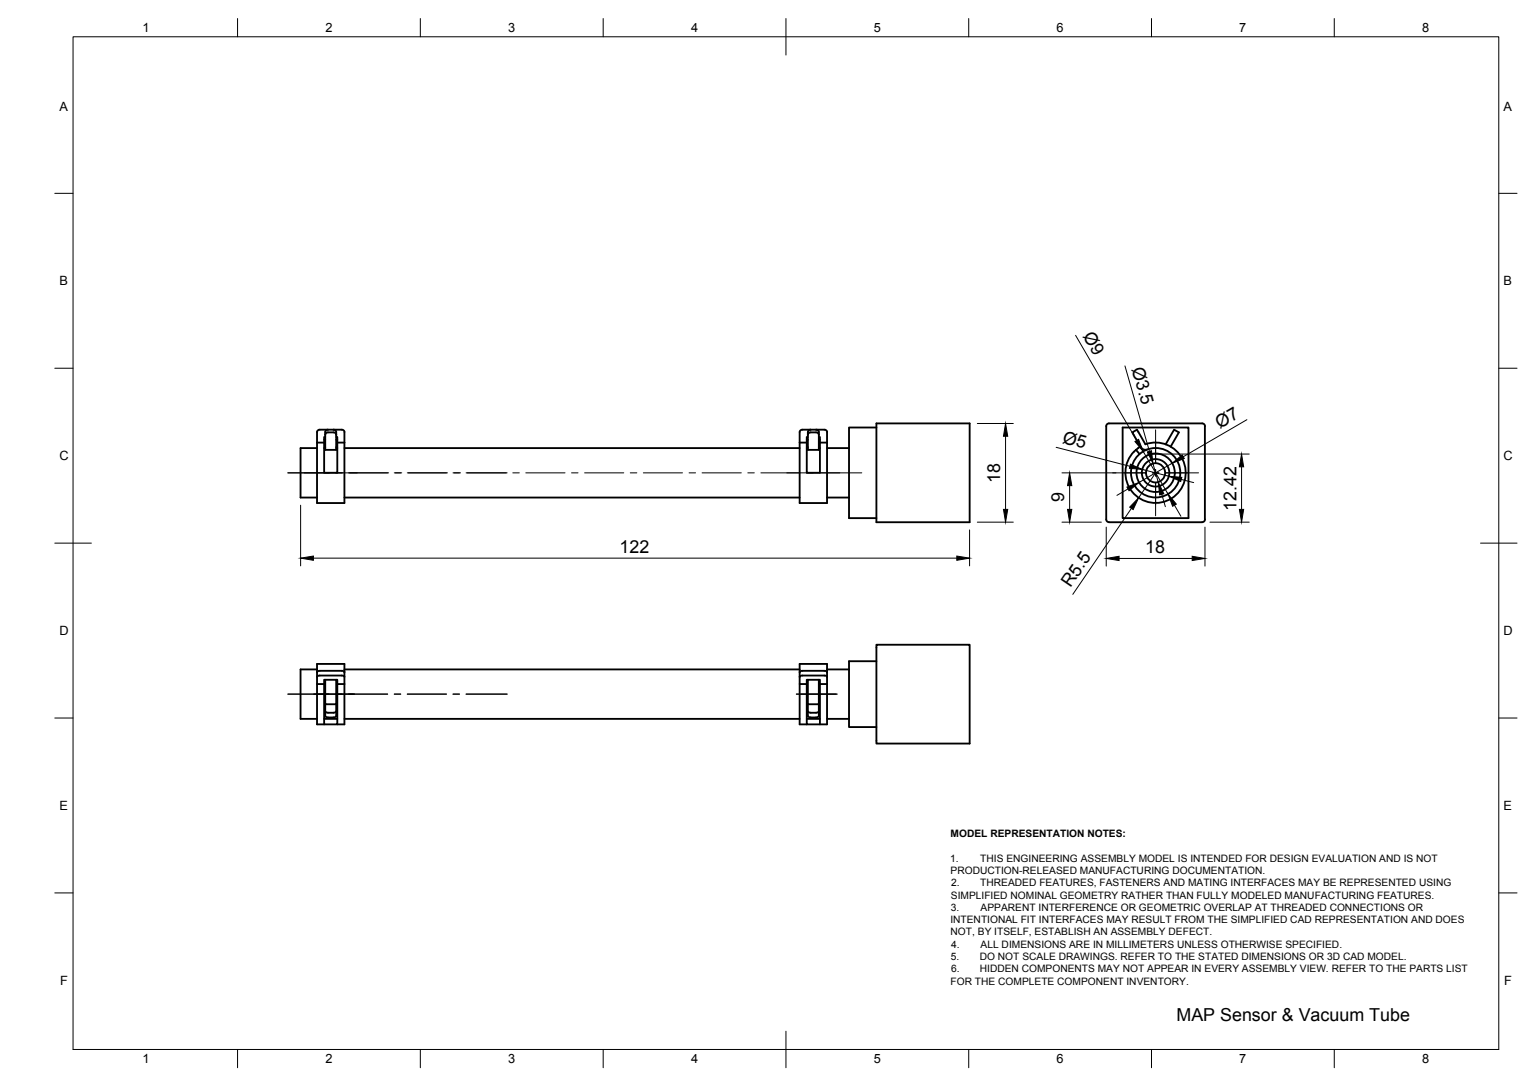
ISO-10303-21;
HEADER;
/* Generated by software containing ST-Developer
 * from STEP Tools, Inc. (www.steptools.com) 
 */

FILE_DESCRIPTION(
/* description */ ('STEP AP214'),
/* implementation_level */ '2;1');

FILE_NAME(
/* name */ 'MAP Sensor & Vacuum Tube.step',
/* time_stamp */ '2026-10-07T12:18:07-07:00',
/* author */ (''),
/* organization */ (''),
/* preprocessor_version */ 'ST-DEVELOPER v20.2',
/* originating_system */ 'Autodesk Translation Framework v15.15.0.0',
/* authorisation */ '');

FILE_SCHEMA (('AUTOMOTIVE_DESIGN { 1 0 10303 214 3 1 1 }'));
ENDSEC;

DATA;
#10=MECHANICAL_DESIGN_GEOMETRIC_PRESENTATION_REPRESENTATION('',(#128),#62974);
#104=SHAPE_REPRESENTATION_RELATIONSHIP('SRR','None',#63027,#116);
#116=ADVANCED_BREP_SHAPE_REPRESENTATION('',(#140),#62968);
#128=STYLED_ITEM('',(#63090),#140);
#140=MANIFOLD_SOLID_BREP('Body1',#15198);
#234=FACE_BOUND('',#5113,.T.);
#235=FACE_BOUND('',#5164,.T.);
#236=FACE_BOUND('',#5166,.T.);
#237=FACE_BOUND('',#5176,.T.);
#238=FACE_BOUND('',#5179,.T.);
#239=FACE_BOUND('',#5183,.T.);
#589=PLANE('',#16296);
#590=PLANE('',#16297);
#591=PLANE('',#16298);
#592=PLANE('',#16302);
#593=PLANE('',#16303);
#594=PLANE('',#16306);
#595=PLANE('',#16311);
#596=PLANE('',#16312);
#597=PLANE('',#16313);
#598=PLANE('',#16315);
#599=PLANE('',#16316);
#600=PLANE('',#16320);
#601=PLANE('',#16321);
#602=PLANE('',#16323);
#603=PLANE('',#16324);
#604=PLANE('',#16325);
#605=PLANE('',#16327);
#606=PLANE('',#16329);
#607=PLANE('',#16333);
#608=PLANE('',#16334);
#609=PLANE('',#16336);
#610=PLANE('',#16337);
#611=PLANE('',#16338);
#612=PLANE('',#16340);
#613=PLANE('',#16341);
#614=PLANE('',#16342);
#615=PLANE('',#16344);
#616=PLANE('',#16345);
#617=PLANE('',#16349);
#618=PLANE('',#16350);
#619=PLANE('',#16357);
#620=PLANE('',#16358);
#621=PLANE('',#16360);
#622=PLANE('',#16361);
#623=PLANE('',#16362);
#624=PLANE('',#16363);
#625=PLANE('',#16364);
#626=PLANE('',#16365);
#627=PLANE('',#16366);
#628=PLANE('',#16367);
#629=PLANE('',#16371);
#630=PLANE('',#16375);
#631=PLANE('',#16376);
#632=PLANE('',#16381);
#633=PLANE('',#16383);
#634=PLANE('',#16384);
#635=PLANE('',#16385);
#636=PLANE('',#16386);
#896=B_SPLINE_CURVE_WITH_KNOTS('',3,(#44539,#44540,#44541,#44542,#44543,
#44544,#44545,#44546,#44547,#44548),.UNSPECIFIED.,.F.,.F.,(4,2,2,2,4),(0.22713486148052,
0.24601821426655,0.264901567052579,0.283737456690072,0.302573346327564),
 .UNSPECIFIED.);
#897=B_SPLINE_CURVE_WITH_KNOTS('',3,(#44552,#44553,#44554,#44555,#44556,
#44557,#44558,#44559,#44560,#44561),.UNSPECIFIED.,.F.,.F.,(4,2,2,2,4),(-0.151286623693373,
-0.132450734062243,-0.113614844431112,-0.0947314916401544,-0.0758481388491969),
 .UNSPECIFIED.);
#898=B_SPLINE_CURVE_WITH_KNOTS('',3,(#44593,#44594,#44595,#44596,#44597,
#44598,#44599,#44600,#44601,#44602),.UNSPECIFIED.,.F.,.F.,(4,2,2,2,4),(0.227134861433275,
0.246018214232104,0.264901567030932,0.283737456679245,0.302573346327559),
 .UNSPECIFIED.);
#899=B_SPLINE_CURVE_WITH_KNOTS('',3,(#44606,#44607,#44608,#44609,#44610,
#44611,#44612,#44613,#44614,#44615),.UNSPECIFIED.,.F.,.F.,(4,2,2,2,4),(-0.151286623693374,
-0.132450734061232,-0.113614844429089,-0.0947314916371198,-0.0758481388451503),
 .UNSPECIFIED.);
#900=B_SPLINE_CURVE_WITH_KNOTS('',3,(#44623,#44624,#44625,#44626,#44627,
#44628,#44629,#44630,#44631,#44632),.UNSPECIFIED.,.F.,.F.,(4,2,2,2,4),(-0.075438484844178,
-0.0565551320532202,-0.0376717792622623,-0.0188358896311301,2.13717932240343E-15),
 .UNSPECIFIED.);
#901=B_SPLINE_CURVE_WITH_KNOTS('',3,(#44636,#44637,#44638,#44639,#44640,
#44641,#44642,#44643,#44644,#44645),.UNSPECIFIED.,.F.,.F.,(4,2,2,2,4),(1.23169706186427E-15,
0.0188358896365198,0.0376717792730385,0.056555132060041,0.0754384848470435),
 .UNSPECIFIED.);
#902=B_SPLINE_CURVE_WITH_KNOTS('',3,(#44665,#44666,#44667,#44668,#44669,
#44670,#44671,#44672,#44673,#44674),.UNSPECIFIED.,.F.,.F.,(4,2,2,2,4),(-0.075438484902782,
-0.0565551320981278,-0.0376717792934735,-0.0188358896467368,0.),
 .UNSPECIFIED.);
#903=B_SPLINE_CURVE_WITH_KNOTS('',3,(#44678,#44679,#44680,#44681,#44682,
#44683,#44684,#44685,#44686,#44687),.UNSPECIFIED.,.F.,.F.,(4,2,2,2,4),(-2.21579007906029E-15,
0.01883588963867,0.0376717792773423,0.0565551320645541,0.0754384848517659),
 .UNSPECIFIED.);
#904=B_SPLINE_CURVE_WITH_KNOTS('',3,(#44704,#44705,#44706,#44707,#44708,
#44709,#44710,#44711,#44712,#44713),.UNSPECIFIED.,.F.,.F.,(4,2,2,2,4),(0.226757476774398,
0.245624555668826,0.264491634563253,0.283327009974748,0.302162385386242),
 .UNSPECIFIED.);
#905=B_SPLINE_CURVE_WITH_KNOTS('',3,(#44717,#44718,#44719,#44720,#44721,
#44722,#44723,#44724,#44725,#44726),.UNSPECIFIED.,.F.,.F.,(4,2,2,2,4),(-0.15108117139346,
-0.132245795981966,-0.113410420570472,-0.0945433416760444,-0.0756762627816166),
 .UNSPECIFIED.);
#906=B_SPLINE_CURVE_WITH_KNOTS('',3,(#44734,#44735,#44736,#44737,#44738,
#44739,#44740,#44741,#44742,#44743),.UNSPECIFIED.,.F.,.F.,(4,2,2,2,4),(-0.226486122604629,
-0.207619043710201,-0.188751964815772,-0.169916589404278,-0.151081213992783),
 .UNSPECIFIED.);
#907=B_SPLINE_CURVE_WITH_KNOTS('',3,(#44747,#44748,#44749,#44750,#44751,
#44752,#44753,#44754,#44755,#44756),.UNSPECIFIED.,.F.,.F.,(4,2,2,2,4),(0.151081213992781,
0.169916589404275,0.18875196481577,0.207619043710198,0.226486122604627),
 .UNSPECIFIED.);
#908=B_SPLINE_CURVE_WITH_KNOTS('',3,(#44765,#44766,#44767,#44768,#44769,
#44770,#44771,#44772,#44773,#44774),.UNSPECIFIED.,.F.,.F.,(4,2,2,2,4),(0.226757476774397,
0.245624555668825,0.264491634563252,0.283327009974748,0.302162385386243),
 .UNSPECIFIED.);
#909=B_SPLINE_CURVE_WITH_KNOTS('',3,(#44778,#44779,#44780,#44781,#44782,
#44783,#44784,#44785,#44786,#44787),.UNSPECIFIED.,.F.,.F.,(4,2,2,2,4),(-0.151081213992782,
-0.132245838581287,-0.113410463169793,-0.0945433842753652,-0.0756763053809372),
 .UNSPECIFIED.);
#910=B_SPLINE_CURVE_WITH_KNOTS('',3,(#44795,#44796,#44797,#44798,#44799,
#44800,#44801,#44802,#44803,#44804),.UNSPECIFIED.,.F.,.F.,(4,2,2,2,4),(-0.226486080005305,
-0.207619001110877,-0.188751922216448,-0.169916546804955,-0.151081171393461),
 .UNSPECIFIED.);
#911=B_SPLINE_CURVE_WITH_KNOTS('',3,(#44808,#44809,#44810,#44811,#44812,
#44813,#44814,#44815,#44816,#44817),.UNSPECIFIED.,.F.,.F.,(4,2,2,2,4),(0.151081171393462,
0.169916546804955,0.188751922216448,0.207619001110876,0.226486080005304),
 .UNSPECIFIED.);
#1803=LINE('',#44535,#2996);
#1804=LINE('',#44550,#2997);
#1805=LINE('',#44565,#2998);
#1806=LINE('',#44570,#2999);
#1807=LINE('',#44575,#3000);
#1808=LINE('',#44579,#3001);
#1809=LINE('',#44584,#3002);
#1810=LINE('',#44589,#3003);
#1811=LINE('',#44604,#3004);
#1812=LINE('',#44619,#3005);
#1813=LINE('',#44634,#3006);
#1814=LINE('',#44650,#3007);
#1815=LINE('',#44655,#3008);
#1816=LINE('',#44661,#3009);
#1817=LINE('',#44676,#3010);
#1818=LINE('',#44691,#3011);
#1819=LINE('',#44695,#3012);
#1820=LINE('',#44700,#3013);
#1821=LINE('',#44715,#3014);
#1822=LINE('',#44730,#3015);
#1823=LINE('',#44745,#3016);
#1824=LINE('',#44761,#3017);
#1825=LINE('',#44776,#3018);
#1826=LINE('',#44791,#3019);
#1827=LINE('',#44806,#3020);
#1828=LINE('',#44823,#3021);
#1829=LINE('',#44829,#3022);
#1830=LINE('',#44835,#3023);
#1831=LINE('',#44842,#3024);
#1832=LINE('',#44845,#3025);
#1833=LINE('',#44850,#3026);
#1834=LINE('',#44856,#3027);
#1835=LINE('',#44862,#3028);
#1836=LINE('',#44866,#3029);
#1837=LINE('',#44870,#3030);
#1838=LINE('',#44876,#3031);
#1839=LINE('',#44882,#3032);
#1840=LINE('',#44888,#3033);
#1841=LINE('',#44892,#3034);
#1842=LINE('',#44896,#3035);
#1843=LINE('',#44903,#3036);
#1844=LINE('',#44908,#3037);
#1845=LINE('',#44916,#3038);
#1846=LINE('',#44920,#3039);
#1847=LINE('',#44921,#3040);
#1848=LINE('',#44923,#3041);
#1849=LINE('',#44924,#3042);
#1850=LINE('',#44930,#3043);
#1851=LINE('',#44933,#3044);
#1852=LINE('',#44935,#3045);
#1853=LINE('',#44936,#3046);
#1854=LINE('',#44937,#3047);
#1855=LINE('',#44940,#3048);
#1856=LINE('',#44943,#3049);
#1857=LINE('',#44946,#3050);
#1858=LINE('',#44948,#3051);
#1859=LINE('',#44950,#3052);
#1860=LINE('',#44951,#3053);
#1861=LINE('',#44954,#3054);
#1862=LINE('',#44957,#3055);
#1863=LINE('',#44959,#3056);
#1864=LINE('',#44961,#3057);
#1865=LINE('',#44964,#3058);
#1866=LINE('',#44966,#3059);
#1867=LINE('',#44967,#3060);
#1868=LINE('',#44969,#3061);
#1869=LINE('',#44970,#3062);
#1870=LINE('',#44975,#3063);
#1871=LINE('',#44976,#3064);
#1872=LINE('',#44981,#3065);
#1873=LINE('',#44985,#3066);
#1874=LINE('',#44987,#3067);
#1875=LINE('',#44988,#3068);
#1876=LINE('',#44992,#3069);
#1877=LINE('',#44994,#3070);
#1878=LINE('',#44995,#3071);
#1879=LINE('',#44998,#3072);
#1880=LINE('',#45000,#3073);
#1881=LINE('',#45001,#3074);
#1882=LINE('',#45003,#3075);
#1883=LINE('',#45006,#3076);
#1884=LINE('',#45010,#3077);
#1885=LINE('',#45011,#3078);
#1886=LINE('',#45017,#3079);
#1887=LINE('',#45020,#3080);
#1888=LINE('',#45023,#3081);
#1889=LINE('',#45025,#3082);
#1890=LINE('',#45026,#3083);
#1891=LINE('',#45030,#3084);
#1892=LINE('',#45032,#3085);
#1893=LINE('',#45034,#3086);
#1894=LINE('',#45035,#3087);
#1895=LINE('',#45036,#3088);
#1896=LINE('',#45039,#3089);
#1897=LINE('',#45041,#3090);
#1898=LINE('',#45042,#3091);
#1899=LINE('',#45044,#3092);
#1900=LINE('',#45047,#3093);
#1901=LINE('',#45049,#3094);
#1902=LINE('',#45050,#3095);
#1903=LINE('',#45052,#3096);
#1904=LINE('',#45053,#3097);
#1905=LINE('',#45055,#3098);
#1906=LINE('',#45059,#3099);
#1907=LINE('',#45060,#3100);
#1908=LINE('',#45062,#3101);
#1909=LINE('',#45063,#3102);
#1910=LINE('',#45069,#3103);
#1911=LINE('',#45072,#3104);
#1912=LINE('',#45074,#3105);
#1913=LINE('',#45075,#3106);
#1914=LINE('',#45076,#3107);
#1915=LINE('',#45079,#3108);
#1916=LINE('',#45082,#3109);
#1917=LINE('',#45086,#3110);
#1918=LINE('',#45089,#3111);
#1919=LINE('',#45091,#3112);
#1920=LINE('',#45094,#3113);
#1921=LINE('',#45095,#3114);
#1922=LINE('',#45106,#3115);
#1923=LINE('',#45108,#3116);
#1924=LINE('',#45110,#3117);
#1925=LINE('',#45111,#3118);
#1926=LINE('',#45114,#3119);
#1927=LINE('',#45116,#3120);
#1928=LINE('',#45117,#3121);
#1929=LINE('',#45121,#3122);
#1930=LINE('',#45123,#3123);
#1931=LINE('',#45125,#3124);
#1932=LINE('',#45126,#3125);
#1933=LINE('',#45131,#3126);
#1934=LINE('',#45135,#3127);
#1935=LINE('',#45137,#3128);
#1936=LINE('',#45138,#3129);
#1937=LINE('',#45143,#3130);
#1938=LINE('',#45147,#3131);
#1939=LINE('',#45149,#3132);
#1940=LINE('',#45150,#3133);
#1941=LINE('',#45155,#3134);
#1942=LINE('',#45159,#3135);
#1943=LINE('',#45163,#3136);
#1944=LINE('',#45166,#3137);
#1945=LINE('',#45167,#3138);
#1946=LINE('',#45169,#3139);
#1947=LINE('',#45172,#3140);
#1948=LINE('',#45173,#3141);
#1949=LINE('',#45175,#3142);
#2996=VECTOR('',#19460,4.5);
#2997=VECTOR('',#19463,1000.);
#2998=VECTOR('',#19466,4.5);
#2999=VECTOR('',#19471,1000.);
#3000=VECTOR('',#19476,4.5);
#3001=VECTOR('',#19479,1000.);
#3002=VECTOR('',#19484,1000.);
#3003=VECTOR('',#19489,4.5);
#3004=VECTOR('',#19492,1000.);
#3005=VECTOR('',#19495,4.5);
#3006=VECTOR('',#19498,1000.);
#3007=VECTOR('',#19503,1000.);
#3008=VECTOR('',#19508,1000.);
#3009=VECTOR('',#19515,4.5);
#3010=VECTOR('',#19518,1000.);
#3011=VECTOR('',#19521,4.5);
#3012=VECTOR('',#19524,1000.);
#3013=VECTOR('',#19529,5.5);
#3014=VECTOR('',#19532,1000.);
#3015=VECTOR('',#19535,1000.);
#3016=VECTOR('',#19538,1000.);
#3017=VECTOR('',#19543,5.5);
#3018=VECTOR('',#19546,1000.);
#3019=VECTOR('',#19549,1000.);
#3020=VECTOR('',#19552,1000.);
#3021=VECTOR('',#19559,2.);
#3022=VECTOR('',#19566,2.5);
#3023=VECTOR('',#19573,1.75);
#3024=VECTOR('',#19580,1000.);
#3025=VECTOR('',#19583,1000.);
#3026=VECTOR('',#19588,1000.);
#3027=VECTOR('',#19595,1000.);
#3028=VECTOR('',#19602,1000.);
#3029=VECTOR('',#19605,1000.);
#3030=VECTOR('',#19608,1000.);
#3031=VECTOR('',#19615,1000.);
#3032=VECTOR('',#19622,1000.);
#3033=VECTOR('',#19629,1000.);
#3034=VECTOR('',#19632,1000.);
#3035=VECTOR('',#19635,1000.);
#3036=VECTOR('',#19644,1000.);
#3037=VECTOR('',#19649,3.5);
#3038=VECTOR('',#19660,1000.);
#3039=VECTOR('',#19667,1000.);
#3040=VECTOR('',#19668,1000.);
#3041=VECTOR('',#19671,1000.);
#3042=VECTOR('',#19672,1000.);
#3043=VECTOR('',#19677,1000.);
#3044=VECTOR('',#19680,1000.);
#3045=VECTOR('',#19683,1000.);
#3046=VECTOR('',#19684,1000.);
#3047=VECTOR('',#19685,1000.);
#3048=VECTOR('',#19688,1000.);
#3049=VECTOR('',#19691,1000.);
#3050=VECTOR('',#19696,1000.);
#3051=VECTOR('',#19697,1000.);
#3052=VECTOR('',#19698,1000.);
#3053=VECTOR('',#19699,1000.);
#3054=VECTOR('',#19702,1000.);
#3055=VECTOR('',#19705,1000.);
#3056=VECTOR('',#19708,1000.);
#3057=VECTOR('',#19711,1000.);
#3058=VECTOR('',#19714,1000.);
#3059=VECTOR('',#19715,1000.);
#3060=VECTOR('',#19716,1000.);
#3061=VECTOR('',#19719,1000.);
#3062=VECTOR('',#19720,1000.);
#3063=VECTOR('',#19729,1000.);
#3064=VECTOR('',#19730,1000.);
#3065=VECTOR('',#19735,1000.);
#3066=VECTOR('',#19740,1000.);
#3067=VECTOR('',#19741,1000.);
#3068=VECTOR('',#19742,1000.);
#3069=VECTOR('',#19747,1000.);
#3070=VECTOR('',#19748,1000.);
#3071=VECTOR('',#19749,1000.);
#3072=VECTOR('',#19752,1000.);
#3073=VECTOR('',#19753,1000.);
#3074=VECTOR('',#19754,1000.);
#3075=VECTOR('',#19757,1000.);
#3076=VECTOR('',#19762,1000.);
#3077=VECTOR('',#19769,1000.);
#3078=VECTOR('',#19770,1000.);
#3079=VECTOR('',#19775,1000.);
#3080=VECTOR('',#19778,1000.);
#3081=VECTOR('',#19781,1000.);
#3082=VECTOR('',#19782,1000.);
#3083=VECTOR('',#19783,1000.);
#3084=VECTOR('',#19788,1000.);
#3085=VECTOR('',#19789,1000.);
#3086=VECTOR('',#19790,1000.);
#3087=VECTOR('',#19791,1000.);
#3088=VECTOR('',#19792,1000.);
#3089=VECTOR('',#19795,1000.);
#3090=VECTOR('',#19796,1000.);
#3091=VECTOR('',#19797,1000.);
#3092=VECTOR('',#19800,1000.);
#3093=VECTOR('',#19803,1000.);
#3094=VECTOR('',#19806,1000.);
#3095=VECTOR('',#19807,1000.);
#3096=VECTOR('',#19810,1000.);
#3097=VECTOR('',#19811,1000.);
#3098=VECTOR('',#19814,1000.);
#3099=VECTOR('',#19821,1000.);
#3100=VECTOR('',#19822,1000.);
#3101=VECTOR('',#19825,1000.);
#3102=VECTOR('',#19826,1000.);
#3103=VECTOR('',#19831,1000.);
#3104=VECTOR('',#19834,1000.);
#3105=VECTOR('',#19837,1000.);
#3106=VECTOR('',#19838,1000.);
#3107=VECTOR('',#19839,1000.);
#3108=VECTOR('',#19842,1000.);
#3109=VECTOR('',#19845,1000.);
#3110=VECTOR('',#19850,1000.);
#3111=VECTOR('',#19853,1000.);
#3112=VECTOR('',#19856,1000.);
#3113=VECTOR('',#19861,1000.);
#3114=VECTOR('',#19862,1000.);
#3115=VECTOR('',#19879,1000.);
#3116=VECTOR('',#19880,1000.);
#3117=VECTOR('',#19881,1000.);
#3118=VECTOR('',#19882,1000.);
#3119=VECTOR('',#19885,1000.);
#3120=VECTOR('',#19886,1000.);
#3121=VECTOR('',#19887,1000.);
#3122=VECTOR('',#19890,1000.);
#3123=VECTOR('',#19891,1000.);
#3124=VECTOR('',#19892,1000.);
#3125=VECTOR('',#19893,1000.);
#3126=VECTOR('',#19898,1000.);
#3127=VECTOR('',#19903,1000.);
#3128=VECTOR('',#19904,1000.);
#3129=VECTOR('',#19905,1000.);
#3130=VECTOR('',#19910,1000.);
#3131=VECTOR('',#19915,1000.);
#3132=VECTOR('',#19916,1000.);
#3133=VECTOR('',#19917,1000.);
#3134=VECTOR('',#19922,1000.);
#3135=VECTOR('',#19927,1000.);
#3136=VECTOR('',#19932,1000.);
#3137=VECTOR('',#19935,1000.);
#3138=VECTOR('',#19936,1000.);
#3139=VECTOR('',#19939,1000.);
#3140=VECTOR('',#19942,1000.);
#3141=VECTOR('',#19943,1000.);
#3142=VECTOR('',#19946,1000.);
#3547=CYLINDRICAL_SURFACE('',#16215,4.5);
#3548=CYLINDRICAL_SURFACE('',#16221,4.5);
#3549=CYLINDRICAL_SURFACE('',#16226,4.5);
#3550=CYLINDRICAL_SURFACE('',#16235,4.5);
#3551=CYLINDRICAL_SURFACE('',#16241,5.5);
#3552=CYLINDRICAL_SURFACE('',#16246,5.5);
#3553=CYLINDRICAL_SURFACE('',#16251,2.);
#3554=CYLINDRICAL_SURFACE('',#16254,2.5);
#3555=CYLINDRICAL_SURFACE('',#16257,1.75);
#3556=CYLINDRICAL_SURFACE('',#16260,1.);
#3557=CYLINDRICAL_SURFACE('',#16263,1.);
#3558=CYLINDRICAL_SURFACE('',#16266,1.);
#3559=CYLINDRICAL_SURFACE('',#16269,5.5);
#3560=CYLINDRICAL_SURFACE('',#16274,1.);
#3561=CYLINDRICAL_SURFACE('',#16277,1.);
#3562=CYLINDRICAL_SURFACE('',#16280,5.5);
#3563=CYLINDRICAL_SURFACE('',#16285,1.);
#3564=CYLINDRICAL_SURFACE('',#16288,3.5);
#3565=CYLINDRICAL_SURFACE('',#16291,4.5);
#3566=CYLINDRICAL_SURFACE('',#16299,0.5);
#3567=CYLINDRICAL_SURFACE('',#16305,0.500000000000001);
#3568=CYLINDRICAL_SURFACE('',#16307,0.5);
#3569=CYLINDRICAL_SURFACE('',#16309,0.500000000000001);
#3570=CYLINDRICAL_SURFACE('',#16310,0.500000000000001);
#3571=CYLINDRICAL_SURFACE('',#16314,0.500000000000001);
#3572=CYLINDRICAL_SURFACE('',#16317,0.5);
#3573=CYLINDRICAL_SURFACE('',#16328,0.5);
#3574=CYLINDRICAL_SURFACE('',#16330,0.5);
#3575=CYLINDRICAL_SURFACE('',#16343,0.5);
#3576=CYLINDRICAL_SURFACE('',#16346,0.5);
#3577=CYLINDRICAL_SURFACE('',#16352,0.5);
#3578=CYLINDRICAL_SURFACE('',#16353,0.5);
#3579=CYLINDRICAL_SURFACE('',#16355,0.5);
#3580=CYLINDRICAL_SURFACE('',#16356,0.5);
#3581=CYLINDRICAL_SURFACE('',#16359,0.5);
#3582=CYLINDRICAL_SURFACE('',#16368,0.500000000000002);
#3583=CYLINDRICAL_SURFACE('',#16372,0.500000000000002);
#3584=CYLINDRICAL_SURFACE('',#16379,0.500000000000002);
#3585=CYLINDRICAL_SURFACE('',#16387,0.500000000000002);
#4186=FACE_OUTER_BOUND('',#5093,.T.);
#4187=FACE_OUTER_BOUND('',#5094,.T.);
#4188=FACE_OUTER_BOUND('',#5095,.T.);
#4189=FACE_OUTER_BOUND('',#5096,.T.);
#4190=FACE_OUTER_BOUND('',#5097,.T.);
#4191=FACE_OUTER_BOUND('',#5098,.T.);
#4192=FACE_OUTER_BOUND('',#5099,.T.);
#4193=FACE_OUTER_BOUND('',#5100,.T.);
#4194=FACE_OUTER_BOUND('',#5101,.T.);
#4195=FACE_OUTER_BOUND('',#5102,.T.);
#4196=FACE_OUTER_BOUND('',#5103,.T.);
#4197=FACE_OUTER_BOUND('',#5104,.T.);
#4198=FACE_OUTER_BOUND('',#5105,.T.);
#4199=FACE_OUTER_BOUND('',#5106,.T.);
#4200=FACE_OUTER_BOUND('',#5107,.T.);
#4201=FACE_OUTER_BOUND('',#5108,.T.);
#4202=FACE_OUTER_BOUND('',#5109,.T.);
#4203=FACE_OUTER_BOUND('',#5110,.T.);
#4204=FACE_OUTER_BOUND('',#5111,.T.);
#4205=FACE_OUTER_BOUND('',#5112,.T.);
#4206=FACE_OUTER_BOUND('',#5114,.T.);
#4207=FACE_OUTER_BOUND('',#5115,.T.);
#4208=FACE_OUTER_BOUND('',#5116,.T.);
#4209=FACE_OUTER_BOUND('',#5117,.T.);
#4210=FACE_OUTER_BOUND('',#5118,.T.);
#4211=FACE_OUTER_BOUND('',#5119,.T.);
#4212=FACE_OUTER_BOUND('',#5120,.T.);
#4213=FACE_OUTER_BOUND('',#5121,.T.);
#4214=FACE_OUTER_BOUND('',#5122,.T.);
#4215=FACE_OUTER_BOUND('',#5123,.T.);
#4216=FACE_OUTER_BOUND('',#5124,.T.);
#4217=FACE_OUTER_BOUND('',#5125,.T.);
#4218=FACE_OUTER_BOUND('',#5126,.T.);
#4219=FACE_OUTER_BOUND('',#5127,.T.);
#4220=FACE_OUTER_BOUND('',#5128,.T.);
#4221=FACE_OUTER_BOUND('',#5129,.T.);
#4222=FACE_OUTER_BOUND('',#5130,.T.);
#4223=FACE_OUTER_BOUND('',#5131,.T.);
#4224=FACE_OUTER_BOUND('',#5132,.T.);
#4225=FACE_OUTER_BOUND('',#5133,.T.);
#4226=FACE_OUTER_BOUND('',#5134,.T.);
#4227=FACE_OUTER_BOUND('',#5135,.T.);
#4228=FACE_OUTER_BOUND('',#5136,.T.);
#4229=FACE_OUTER_BOUND('',#5137,.T.);
#4230=FACE_OUTER_BOUND('',#5138,.T.);
#4231=FACE_OUTER_BOUND('',#5139,.T.);
#4232=FACE_OUTER_BOUND('',#5140,.T.);
#4233=FACE_OUTER_BOUND('',#5141,.T.);
#4234=FACE_OUTER_BOUND('',#5142,.T.);
#4235=FACE_OUTER_BOUND('',#5143,.T.);
#4236=FACE_OUTER_BOUND('',#5144,.T.);
#4237=FACE_OUTER_BOUND('',#5145,.T.);
#4238=FACE_OUTER_BOUND('',#5146,.T.);
#4239=FACE_OUTER_BOUND('',#5147,.T.);
#4240=FACE_OUTER_BOUND('',#5148,.T.);
#4241=FACE_OUTER_BOUND('',#5149,.T.);
#4242=FACE_OUTER_BOUND('',#5150,.T.);
#4243=FACE_OUTER_BOUND('',#5151,.T.);
#4244=FACE_OUTER_BOUND('',#5152,.T.);
#4245=FACE_OUTER_BOUND('',#5153,.T.);
#4246=FACE_OUTER_BOUND('',#5154,.T.);
#4247=FACE_OUTER_BOUND('',#5155,.T.);
#4248=FACE_OUTER_BOUND('',#5156,.T.);
#4249=FACE_OUTER_BOUND('',#5157,.T.);
#4250=FACE_OUTER_BOUND('',#5158,.T.);
#4251=FACE_OUTER_BOUND('',#5159,.T.);
#4252=FACE_OUTER_BOUND('',#5160,.T.);
#4253=FACE_OUTER_BOUND('',#5161,.T.);
#4254=FACE_OUTER_BOUND('',#5162,.T.);
#4255=FACE_OUTER_BOUND('',#5163,.T.);
#4256=FACE_OUTER_BOUND('',#5165,.T.);
#4257=FACE_OUTER_BOUND('',#5167,.T.);
#4258=FACE_OUTER_BOUND('',#5168,.T.);
#4259=FACE_OUTER_BOUND('',#5169,.T.);
#4260=FACE_OUTER_BOUND('',#5170,.T.);
#4261=FACE_OUTER_BOUND('',#5171,.T.);
#4262=FACE_OUTER_BOUND('',#5172,.T.);
#4263=FACE_OUTER_BOUND('',#5173,.T.);
#4264=FACE_OUTER_BOUND('',#5174,.T.);
#4265=FACE_OUTER_BOUND('',#5175,.T.);
#4266=FACE_OUTER_BOUND('',#5177,.T.);
#4267=FACE_OUTER_BOUND('',#5178,.T.);
#4268=FACE_OUTER_BOUND('',#5180,.T.);
#4269=FACE_OUTER_BOUND('',#5181,.T.);
#4270=FACE_OUTER_BOUND('',#5182,.T.);
#4271=FACE_OUTER_BOUND('',#5184,.T.);
#4272=FACE_OUTER_BOUND('',#5185,.T.);
#5093=EDGE_LOOP('',(#12327,#12328,#12329,#12330,#12331,#12332,#12333,#12334,
#12335,#12336,#12337,#12338));
#5094=EDGE_LOOP('',(#12339,#12340,#12341,#12342,#12343,#12344,#12345,#12346));
#5095=EDGE_LOOP('',(#12347,#12348,#12349,#12350,#12351,#12352,#12353,#12354,
#12355,#12356,#12357,#12358,#12359,#12360,#12361,#12362,#12363,#12364,#12365,
#12366));
#5096=EDGE_LOOP('',(#12367,#12368,#12369,#12370,#12371,#12372,#12373,#12374,
#12375,#12376,#12377,#12378));
#5097=EDGE_LOOP('',(#12379,#12380,#12381,#12382,#12383,#12384,#12385,#12386,
#12387,#12388,#12389,#12390));
#5098=EDGE_LOOP('',(#12391,#12392,#12393,#12394,#12395,#12396,#12397,#12398,
#12399,#12400,#12401,#12402));
#5099=EDGE_LOOP('',(#12403,#12404,#12405,#12406));
#5100=EDGE_LOOP('',(#12407,#12408,#12409,#12410));
#5101=EDGE_LOOP('',(#12411,#12412,#12413,#12414));
#5102=EDGE_LOOP('',(#12415,#12416,#12417,#12418));
#5103=EDGE_LOOP('',(#12419,#12420,#12421,#12422));
#5104=EDGE_LOOP('',(#12423,#12424,#12425,#12426));
#5105=EDGE_LOOP('',(#12427,#12428,#12429,#12430,#12431,#12432,#12433,#12434));
#5106=EDGE_LOOP('',(#12435,#12436,#12437,#12438));
#5107=EDGE_LOOP('',(#12439,#12440,#12441,#12442));
#5108=EDGE_LOOP('',(#12443,#12444,#12445,#12446,#12447,#12448,#12449,#12450));
#5109=EDGE_LOOP('',(#12451,#12452,#12453,#12454));
#5110=EDGE_LOOP('',(#12455,#12456,#12457,#12458));
#5111=EDGE_LOOP('',(#12459,#12460,#12461,#12462,#12463,#12464,#12465,#12466));
#5112=EDGE_LOOP('',(#12467));
#5113=EDGE_LOOP('',(#12468));
#5114=EDGE_LOOP('',(#12469,#12470,#12471,#12472));
#5115=EDGE_LOOP('',(#12473,#12474,#12475,#12476));
#5116=EDGE_LOOP('',(#12477,#12478,#12479,#12480));
#5117=EDGE_LOOP('',(#12481,#12482,#12483,#12484,#12485,#12486,#12487,#12488));
#5118=EDGE_LOOP('',(#12489,#12490,#12491,#12492,#12493,#12494));
#5119=EDGE_LOOP('',(#12495,#12496,#12497,#12498));
#5120=EDGE_LOOP('',(#12499,#12500,#12501,#12502,#12503,#12504,#12505,#12506,
#12507));
#5121=EDGE_LOOP('',(#12508,#12509,#12510,#12511));
#5122=EDGE_LOOP('',(#12512,#12513,#12514,#12515));
#5123=EDGE_LOOP('',(#12516,#12517,#12518,#12519));
#5124=EDGE_LOOP('',(#12520,#12521,#12522,#12523,#12524,#12525,#12526,#12527,
#12528));
#5125=EDGE_LOOP('',(#12529,#12530,#12531,#12532,#12533,#12534));
#5126=EDGE_LOOP('',(#12535,#12536,#12537,#12538,#12539,#12540,#12541,#12542));
#5127=EDGE_LOOP('',(#12543,#12544,#12545,#12546));
#5128=EDGE_LOOP('',(#12547,#12548,#12549,#12550));
#5129=EDGE_LOOP('',(#12551,#12552,#12553,#12554));
#5130=EDGE_LOOP('',(#12555,#12556,#12557,#12558));
#5131=EDGE_LOOP('',(#12559,#12560,#12561,#12562));
#5132=EDGE_LOOP('',(#12563,#12564,#12565,#12566,#12567,#12568,#12569,#12570,
#12571,#12572));
#5133=EDGE_LOOP('',(#12573,#12574,#12575,#12576));
#5134=EDGE_LOOP('',(#12577,#12578,#12579,#12580,#12581,#12582,#12583,#12584));
#5135=EDGE_LOOP('',(#12585,#12586,#12587,#12588,#12589,#12590,#12591,#12592,
#12593,#12594));
#5136=EDGE_LOOP('',(#12595,#12596,#12597,#12598,#12599,#12600,#12601,#12602));
#5137=EDGE_LOOP('',(#12603,#12604,#12605,#12606));
#5138=EDGE_LOOP('',(#12607,#12608,#12609,#12610));
#5139=EDGE_LOOP('',(#12611,#12612,#12613,#12614));
#5140=EDGE_LOOP('',(#12615,#12616,#12617,#12618));
#5141=EDGE_LOOP('',(#12619,#12620,#12621,#12622,#12623,#12624,#12625,#12626,
#12627,#12628));
#5142=EDGE_LOOP('',(#12629,#12630,#12631,#12632));
#5143=EDGE_LOOP('',(#12633,#12634,#12635,#12636,#12637,#12638,#12639,#12640));
#5144=EDGE_LOOP('',(#12641,#12642,#12643,#12644,#12645,#12646,#12647,#12648,
#12649,#12650));
#5145=EDGE_LOOP('',(#12651,#12652,#12653,#12654,#12655,#12656,#12657,#12658,
#12659));
#5146=EDGE_LOOP('',(#12660,#12661,#12662,#12663,#12664,#12665,#12666,#12667,
#12668));
#5147=EDGE_LOOP('',(#12669,#12670,#12671,#12672,#12673,#12674,#12675,#12676));
#5148=EDGE_LOOP('',(#12677,#12678,#12679,#12680));
#5149=EDGE_LOOP('',(#12681,#12682,#12683,#12684));
#5150=EDGE_LOOP('',(#12685,#12686,#12687,#12688));
#5151=EDGE_LOOP('',(#12689,#12690,#12691,#12692));
#5152=EDGE_LOOP('',(#12693,#12694,#12695,#12696,#12697,#12698,#12699,#12700));
#5153=EDGE_LOOP('',(#12701,#12702,#12703,#12704,#12705,#12706));
#5154=EDGE_LOOP('',(#12707,#12708,#12709,#12710));
#5155=EDGE_LOOP('',(#12711,#12712,#12713,#12714));
#5156=EDGE_LOOP('',(#12715,#12716,#12717,#12718));
#5157=EDGE_LOOP('',(#12719,#12720,#12721,#12722));
#5158=EDGE_LOOP('',(#12723,#12724,#12725,#12726,#12727,#12728));
#5159=EDGE_LOOP('',(#12729,#12730,#12731,#12732,#12733,#12734,#12735,#12736));
#5160=EDGE_LOOP('',(#12737,#12738,#12739,#12740));
#5161=EDGE_LOOP('',(#12741,#12742,#12743,#12744));
#5162=EDGE_LOOP('',(#12745));
#5163=EDGE_LOOP('',(#12746));
#5164=EDGE_LOOP('',(#12747));
#5165=EDGE_LOOP('',(#12748));
#5166=EDGE_LOOP('',(#12749));
#5167=EDGE_LOOP('',(#12750));
#5168=EDGE_LOOP('',(#12751,#12752,#12753,#12754));
#5169=EDGE_LOOP('',(#12755,#12756,#12757,#12758));
#5170=EDGE_LOOP('',(#12759,#12760,#12761,#12762));
#5171=EDGE_LOOP('',(#12763,#12764,#12765,#12766));
#5172=EDGE_LOOP('',(#12767,#12768,#12769,#12770));
#5173=EDGE_LOOP('',(#12771,#12772,#12773,#12774));
#5174=EDGE_LOOP('',(#12775,#12776,#12777,#12778));
#5175=EDGE_LOOP('',(#12779,#12780,#12781,#12782,#12783,#12784,#12785,#12786));
#5176=EDGE_LOOP('',(#12787));
#5177=EDGE_LOOP('',(#12788,#12789,#12790,#12791));
#5178=EDGE_LOOP('',(#12792,#12793,#12794,#12795,#12796,#12797,#12798,#12799));
#5179=EDGE_LOOP('',(#12800,#12801,#12802,#12803));
#5180=EDGE_LOOP('',(#12804,#12805,#12806,#12807));
#5181=EDGE_LOOP('',(#12808,#12809,#12810,#12811));
#5182=EDGE_LOOP('',(#12812,#12813,#12814,#12815));
#5183=EDGE_LOOP('',(#12816));
#5184=EDGE_LOOP('',(#12817,#12818,#12819,#12820));
#5185=EDGE_LOOP('',(#12821,#12822,#12823,#12824));
#5872=CIRCLE('',#16216,4.5);
#5873=CIRCLE('',#16217,4.5);
#5874=CIRCLE('',#16218,4.5);
#5875=CIRCLE('',#16219,4.5);
#5876=CIRCLE('',#16220,4.5);
#5877=CIRCLE('',#16222,4.5);
#5878=CIRCLE('',#16223,4.5);
#5879=CIRCLE('',#16224,4.5);
#5880=CIRCLE('',#16225,4.5);
#5881=CIRCLE('',#16227,4.5);
#5882=CIRCLE('',#16228,4.5);
#5883=CIRCLE('',#16229,4.5);
#5884=CIRCLE('',#16230,4.5);
#5885=CIRCLE('',#16231,4.5);
#5886=CIRCLE('',#16232,4.5);
#5887=CIRCLE('',#16233,4.5);
#5888=CIRCLE('',#16234,4.5);
#5889=CIRCLE('',#16236,4.5);
#5890=CIRCLE('',#16237,4.5);
#5891=CIRCLE('',#16238,4.5);
#5892=CIRCLE('',#16239,4.5);
#5893=CIRCLE('',#16240,4.5);
#5894=CIRCLE('',#16242,5.5);
#5895=CIRCLE('',#16243,5.5);
#5896=CIRCLE('',#16244,5.5);
#5897=CIRCLE('',#16245,5.5);
#5898=CIRCLE('',#16247,5.5);
#5899=CIRCLE('',#16248,5.5);
#5900=CIRCLE('',#16249,5.5);
#5901=CIRCLE('',#16250,5.5);
#5902=CIRCLE('',#16252,2.);
#5903=CIRCLE('',#16253,2.);
#5904=CIRCLE('',#16255,2.5);
#5905=CIRCLE('',#16256,2.5);
#5906=CIRCLE('',#16258,1.75);
#5907=CIRCLE('',#16259,1.75);
#5908=CIRCLE('',#16261,1.);
#5909=CIRCLE('',#16262,1.);
#5910=CIRCLE('',#16264,0.999999999999999);
#5911=CIRCLE('',#16265,1.);
#5912=CIRCLE('',#16267,1.);
#5913=CIRCLE('',#16268,0.999999999999999);
#5914=CIRCLE('',#16270,5.5);
#5915=CIRCLE('',#16271,5.50000000000001);
#5916=CIRCLE('',#16272,5.50000000000001);
#5917=CIRCLE('',#16273,5.5);
#5918=CIRCLE('',#16275,0.999999999999999);
#5919=CIRCLE('',#16276,1.);
#5920=CIRCLE('',#16278,1.);
#5921=CIRCLE('',#16279,0.999999999999999);
#5922=CIRCLE('',#16281,5.5);
#5923=CIRCLE('',#16282,5.50000000000001);
#5924=CIRCLE('',#16283,5.50000000000001);
#5925=CIRCLE('',#16284,5.5);
#5926=CIRCLE('',#16286,1.);
#5927=CIRCLE('',#16287,1.);
#5928=CIRCLE('',#16289,3.5);
#5929=CIRCLE('',#16290,3.5);
#5930=CIRCLE('',#16292,4.5);
#5931=CIRCLE('',#16293,4.5);
#5932=CIRCLE('',#16294,4.5);
#5933=CIRCLE('',#16295,4.5);
#5934=CIRCLE('',#16300,0.5);
#5935=CIRCLE('',#16301,0.5);
#5936=CIRCLE('',#16304,0.5);
#5937=CIRCLE('',#16308,0.5);
#5938=CIRCLE('',#16318,0.5);
#5939=CIRCLE('',#16319,0.5);
#5940=CIRCLE('',#16322,0.5);
#5941=CIRCLE('',#16326,0.5);
#5942=CIRCLE('',#16331,0.5);
#5943=CIRCLE('',#16332,0.5);
#5944=CIRCLE('',#16335,0.5);
#5945=CIRCLE('',#16339,0.5);
#5946=CIRCLE('',#16347,0.5);
#5947=CIRCLE('',#16348,0.5);
#5948=CIRCLE('',#16351,0.5);
#5949=CIRCLE('',#16354,0.5);
#5950=CIRCLE('',#16369,0.500000000000002);
#5951=CIRCLE('',#16370,0.5);
#5952=CIRCLE('',#16373,0.500000000000002);
#5953=CIRCLE('',#16374,0.5);
#5954=CIRCLE('',#16377,0.500000000000002);
#5955=CIRCLE('',#16378,0.500000000000002);
#5956=CIRCLE('',#16380,0.5);
#5957=CIRCLE('',#16382,0.5);
#7010=VERTEX_POINT('',#44533);
#7011=VERTEX_POINT('',#44534);
#7012=VERTEX_POINT('',#44536);
#7013=VERTEX_POINT('',#44538);
#7014=VERTEX_POINT('',#44549);
#7015=VERTEX_POINT('',#44551);
#7016=VERTEX_POINT('',#44562);
#7017=VERTEX_POINT('',#44564);
#7018=VERTEX_POINT('',#44567);
#7019=VERTEX_POINT('',#44569);
#7020=VERTEX_POINT('',#44573);
#7021=VERTEX_POINT('',#44574);
#7022=VERTEX_POINT('',#44576);
#7023=VERTEX_POINT('',#44578);
#7024=VERTEX_POINT('',#44581);
#7025=VERTEX_POINT('',#44583);
#7026=VERTEX_POINT('',#44587);
#7027=VERTEX_POINT('',#44588);
#7028=VERTEX_POINT('',#44590);
#7029=VERTEX_POINT('',#44592);
#7030=VERTEX_POINT('',#44603);
#7031=VERTEX_POINT('',#44605);
#7032=VERTEX_POINT('',#44616);
#7033=VERTEX_POINT('',#44618);
#7034=VERTEX_POINT('',#44620);
#7035=VERTEX_POINT('',#44622);
#7036=VERTEX_POINT('',#44633);
#7037=VERTEX_POINT('',#44635);
#7038=VERTEX_POINT('',#44647);
#7039=VERTEX_POINT('',#44649);
#7040=VERTEX_POINT('',#44652);
#7041=VERTEX_POINT('',#44654);
#7042=VERTEX_POINT('',#44658);
#7043=VERTEX_POINT('',#44660);
#7044=VERTEX_POINT('',#44662);
#7045=VERTEX_POINT('',#44664);
#7046=VERTEX_POINT('',#44675);
#7047=VERTEX_POINT('',#44677);
#7048=VERTEX_POINT('',#44688);
#7049=VERTEX_POINT('',#44690);
#7050=VERTEX_POINT('',#44692);
#7051=VERTEX_POINT('',#44694);
#7052=VERTEX_POINT('',#44698);
#7053=VERTEX_POINT('',#44699);
#7054=VERTEX_POINT('',#44701);
#7055=VERTEX_POINT('',#44703);
#7056=VERTEX_POINT('',#44714);
#7057=VERTEX_POINT('',#44716);
#7058=VERTEX_POINT('',#44727);
#7059=VERTEX_POINT('',#44729);
#7060=VERTEX_POINT('',#44731);
#7061=VERTEX_POINT('',#44733);
#7062=VERTEX_POINT('',#44744);
#7063=VERTEX_POINT('',#44746);
#7064=VERTEX_POINT('',#44759);
#7065=VERTEX_POINT('',#44760);
#7066=VERTEX_POINT('',#44762);
#7067=VERTEX_POINT('',#44764);
#7068=VERTEX_POINT('',#44775);
#7069=VERTEX_POINT('',#44777);
#7070=VERTEX_POINT('',#44788);
#7071=VERTEX_POINT('',#44790);
#7072=VERTEX_POINT('',#44792);
#7073=VERTEX_POINT('',#44794);
#7074=VERTEX_POINT('',#44805);
#7075=VERTEX_POINT('',#44807);
#7076=VERTEX_POINT('',#44820);
#7077=VERTEX_POINT('',#44822);
#7078=VERTEX_POINT('',#44826);
#7079=VERTEX_POINT('',#44828);
#7080=VERTEX_POINT('',#44832);
#7081=VERTEX_POINT('',#44834);
#7082=VERTEX_POINT('',#44838);
#7083=VERTEX_POINT('',#44839);
#7084=VERTEX_POINT('',#44841);
#7085=VERTEX_POINT('',#44843);
#7086=VERTEX_POINT('',#44847);
#7087=VERTEX_POINT('',#44849);
#7088=VERTEX_POINT('',#44853);
#7089=VERTEX_POINT('',#44855);
#7090=VERTEX_POINT('',#44859);
#7091=VERTEX_POINT('',#44861);
#7092=VERTEX_POINT('',#44863);
#7093=VERTEX_POINT('',#44865);
#7094=VERTEX_POINT('',#44867);
#7095=VERTEX_POINT('',#44869);
#7096=VERTEX_POINT('',#44873);
#7097=VERTEX_POINT('',#44875);
#7098=VERTEX_POINT('',#44879);
#7099=VERTEX_POINT('',#44881);
#7100=VERTEX_POINT('',#44885);
#7101=VERTEX_POINT('',#44887);
#7102=VERTEX_POINT('',#44889);
#7103=VERTEX_POINT('',#44891);
#7104=VERTEX_POINT('',#44893);
#7105=VERTEX_POINT('',#44895);
#7106=VERTEX_POINT('',#44899);
#7107=VERTEX_POINT('',#44901);
#7108=VERTEX_POINT('',#44905);
#7109=VERTEX_POINT('',#44907);
#7110=VERTEX_POINT('',#44913);
#7111=VERTEX_POINT('',#44915);
#7112=VERTEX_POINT('',#44926);
#7113=VERTEX_POINT('',#44927);
#7114=VERTEX_POINT('',#44929);
#7115=VERTEX_POINT('',#44931);
#7116=VERTEX_POINT('',#44939);
#7117=VERTEX_POINT('',#44941);
#7118=VERTEX_POINT('',#44947);
#7119=VERTEX_POINT('',#44949);
#7120=VERTEX_POINT('',#44953);
#7121=VERTEX_POINT('',#44955);
#7122=VERTEX_POINT('',#44963);
#7123=VERTEX_POINT('',#44965);
#7124=VERTEX_POINT('',#44978);
#7125=VERTEX_POINT('',#44980);
#7126=VERTEX_POINT('',#44984);
#7127=VERTEX_POINT('',#44986);
#7128=VERTEX_POINT('',#44991);
#7129=VERTEX_POINT('',#44993);
#7130=VERTEX_POINT('',#44997);
#7131=VERTEX_POINT('',#44999);
#7132=VERTEX_POINT('',#45013);
#7133=VERTEX_POINT('',#45014);
#7134=VERTEX_POINT('',#45016);
#7135=VERTEX_POINT('',#45018);
#7136=VERTEX_POINT('',#45022);
#7137=VERTEX_POINT('',#45024);
#7138=VERTEX_POINT('',#45028);
#7139=VERTEX_POINT('',#45031);
#7140=VERTEX_POINT('',#45033);
#7141=VERTEX_POINT('',#45038);
#7142=VERTEX_POINT('',#45040);
#7143=VERTEX_POINT('',#45046);
#7144=VERTEX_POINT('',#45065);
#7145=VERTEX_POINT('',#45066);
#7146=VERTEX_POINT('',#45068);
#7147=VERTEX_POINT('',#45070);
#7148=VERTEX_POINT('',#45078);
#7149=VERTEX_POINT('',#45080);
#7150=VERTEX_POINT('',#45085);
#7151=VERTEX_POINT('',#45087);
#7152=VERTEX_POINT('',#45104);
#7153=VERTEX_POINT('',#45105);
#7154=VERTEX_POINT('',#45107);
#7155=VERTEX_POINT('',#45109);
#7156=VERTEX_POINT('',#45113);
#7157=VERTEX_POINT('',#45115);
#7158=VERTEX_POINT('',#45119);
#7159=VERTEX_POINT('',#45120);
#7160=VERTEX_POINT('',#45122);
#7161=VERTEX_POINT('',#45124);
#7162=VERTEX_POINT('',#45128);
#7163=VERTEX_POINT('',#45130);
#7164=VERTEX_POINT('',#45134);
#7165=VERTEX_POINT('',#45136);
#7166=VERTEX_POINT('',#45140);
#7167=VERTEX_POINT('',#45142);
#7168=VERTEX_POINT('',#45146);
#7169=VERTEX_POINT('',#45148);
#7170=VERTEX_POINT('',#45152);
#7171=VERTEX_POINT('',#45154);
#7172=VERTEX_POINT('',#45158);
#7173=VERTEX_POINT('',#45162);
#7174=VERTEX_POINT('',#45165);
#7175=VERTEX_POINT('',#45171);
#8870=EDGE_CURVE('',#7010,#7011,#1803,.T.);
#8871=EDGE_CURVE('',#7010,#7012,#5872,.T.);
#8872=EDGE_CURVE('',#7012,#7013,#896,.T.);
#8873=EDGE_CURVE('',#7014,#7013,#1804,.T.);
#8874=EDGE_CURVE('',#7014,#7015,#897,.T.);
#8875=EDGE_CURVE('',#7016,#7015,#5873,.T.);
#8876=EDGE_CURVE('',#7016,#7017,#1805,.T.);
#8877=EDGE_CURVE('',#7017,#7017,#5874,.T.);
#8878=EDGE_CURVE('',#7018,#7016,#5875,.T.);
#8879=EDGE_CURVE('',#7018,#7019,#1806,.T.);
#8880=EDGE_CURVE('',#7011,#7019,#5876,.T.);
#8881=EDGE_CURVE('',#7020,#7021,#1807,.T.);
#8882=EDGE_CURVE('',#7022,#7021,#5877,.T.);
#8883=EDGE_CURVE('',#7023,#7022,#1808,.T.);
#8884=EDGE_CURVE('',#7023,#7010,#5878,.T.);
#8885=EDGE_CURVE('',#7024,#7011,#5879,.T.);
#8886=EDGE_CURVE('',#7025,#7024,#1809,.T.);
#8887=EDGE_CURVE('',#7025,#7020,#5880,.T.);
#8888=EDGE_CURVE('',#7026,#7027,#1810,.T.);
#8889=EDGE_CURVE('',#7026,#7028,#5881,.T.);
#8890=EDGE_CURVE('',#7028,#7029,#898,.T.);
#8891=EDGE_CURVE('',#7030,#7029,#1811,.T.);
#8892=EDGE_CURVE('',#7030,#7031,#899,.T.);
#8893=EDGE_CURVE('',#7032,#7031,#5882,.T.);
#8894=EDGE_CURVE('',#7032,#7033,#1812,.T.);
#8895=EDGE_CURVE('',#7033,#7034,#5883,.T.);
#8896=EDGE_CURVE('',#7034,#7035,#900,.T.);
#8897=EDGE_CURVE('',#7035,#7036,#1813,.T.);
#8898=EDGE_CURVE('',#7036,#7037,#901,.T.);
#8899=EDGE_CURVE('',#7021,#7037,#5884,.T.);
#8900=EDGE_CURVE('',#7020,#7038,#5885,.T.);
#8901=EDGE_CURVE('',#7038,#7039,#1814,.T.);
#8902=EDGE_CURVE('',#7039,#7033,#5886,.T.);
#8903=EDGE_CURVE('',#7040,#7032,#5887,.T.);
#8904=EDGE_CURVE('',#7040,#7041,#1815,.T.);
#8905=EDGE_CURVE('',#7027,#7041,#5888,.T.);
#8906=EDGE_CURVE('',#7042,#7042,#5889,.T.);
#8907=EDGE_CURVE('',#7042,#7043,#1816,.T.);
#8908=EDGE_CURVE('',#7043,#7044,#5890,.T.);
#8909=EDGE_CURVE('',#7044,#7045,#902,.T.);
#8910=EDGE_CURVE('',#7045,#7046,#1817,.T.);
#8911=EDGE_CURVE('',#7046,#7047,#903,.T.);
#8912=EDGE_CURVE('',#7048,#7047,#5891,.T.);
#8913=EDGE_CURVE('',#7049,#7048,#1818,.T.);
#8914=EDGE_CURVE('',#7049,#7050,#5892,.T.);
#8915=EDGE_CURVE('',#7050,#7051,#1819,.T.);
#8916=EDGE_CURVE('',#7051,#7043,#5893,.T.);
#8917=EDGE_CURVE('',#7052,#7053,#1820,.T.);
#8918=EDGE_CURVE('',#7052,#7054,#5894,.T.);
#8919=EDGE_CURVE('',#7054,#7055,#904,.T.);
#8920=EDGE_CURVE('',#7056,#7055,#1821,.T.);
#8921=EDGE_CURVE('',#7056,#7057,#905,.T.);
#8922=EDGE_CURVE('',#7058,#7057,#5895,.T.);
#8923=EDGE_CURVE('',#7059,#7058,#1822,.T.);
#8924=EDGE_CURVE('',#7059,#7060,#5896,.T.);
#8925=EDGE_CURVE('',#7060,#7061,#906,.T.);
#8926=EDGE_CURVE('',#7061,#7062,#1823,.T.);
#8927=EDGE_CURVE('',#7062,#7063,#907,.T.);
#8928=EDGE_CURVE('',#7053,#7063,#5897,.T.);
#8929=EDGE_CURVE('',#7064,#7065,#1824,.T.);
#8930=EDGE_CURVE('',#7064,#7066,#5898,.T.);
#8931=EDGE_CURVE('',#7066,#7067,#908,.T.);
#8932=EDGE_CURVE('',#7068,#7067,#1825,.T.);
#8933=EDGE_CURVE('',#7068,#7069,#909,.T.);
#8934=EDGE_CURVE('',#7070,#7069,#5899,.T.);
#8935=EDGE_CURVE('',#7071,#7070,#1826,.T.);
#8936=EDGE_CURVE('',#7071,#7072,#5900,.T.);
#8937=EDGE_CURVE('',#7072,#7073,#910,.T.);
#8938=EDGE_CURVE('',#7073,#7074,#1827,.T.);
#8939=EDGE_CURVE('',#7074,#7075,#911,.T.);
#8940=EDGE_CURVE('',#7065,#7075,#5901,.T.);
#8941=EDGE_CURVE('',#7076,#7076,#5902,.T.);
#8942=EDGE_CURVE('',#7076,#7077,#1828,.T.);
#8943=EDGE_CURVE('',#7077,#7077,#5903,.T.);
#8944=EDGE_CURVE('',#7078,#7078,#5904,.T.);
#8945=EDGE_CURVE('',#7078,#7079,#1829,.T.);
#8946=EDGE_CURVE('',#7079,#7079,#5905,.T.);
#8947=EDGE_CURVE('',#7080,#7080,#5906,.T.);
#8948=EDGE_CURVE('',#7080,#7081,#1830,.T.);
#8949=EDGE_CURVE('',#7081,#7081,#5907,.T.);
#8950=EDGE_CURVE('',#7082,#7083,#5908,.T.);
#8951=EDGE_CURVE('',#7083,#7084,#1831,.T.);
#8952=EDGE_CURVE('',#7085,#7084,#5909,.T.);
#8953=EDGE_CURVE('',#7082,#7085,#1832,.T.);
#8954=EDGE_CURVE('',#7050,#7086,#5910,.T.);
#8955=EDGE_CURVE('',#7086,#7087,#1833,.T.);
#8956=EDGE_CURVE('',#7087,#7051,#5911,.T.);
#8957=EDGE_CURVE('',#7088,#7040,#5912,.T.);
#8958=EDGE_CURVE('',#7088,#7089,#1834,.T.);
#8959=EDGE_CURVE('',#7041,#7089,#5913,.T.);
#8960=EDGE_CURVE('',#7090,#7065,#5914,.T.);
#8961=EDGE_CURVE('',#7090,#7091,#1835,.T.);
#8962=EDGE_CURVE('',#7092,#7091,#5915,.T.);
#8963=EDGE_CURVE('',#7093,#7092,#1836,.T.);
#8964=EDGE_CURVE('',#7093,#7094,#5916,.T.);
#8965=EDGE_CURVE('',#7094,#7095,#1837,.T.);
#8966=EDGE_CURVE('',#7095,#7064,#5917,.T.);
#8967=EDGE_CURVE('',#7038,#7096,#5918,.T.);
#8968=EDGE_CURVE('',#7096,#7097,#1838,.T.);
#8969=EDGE_CURVE('',#7097,#7039,#5919,.T.);
#8970=EDGE_CURVE('',#7098,#7018,#5920,.T.);
#8971=EDGE_CURVE('',#7098,#7099,#1839,.T.);
#8972=EDGE_CURVE('',#7019,#7099,#5921,.T.);
#8973=EDGE_CURVE('',#7100,#7053,#5922,.T.);
#8974=EDGE_CURVE('',#7100,#7101,#1840,.T.);
#8975=EDGE_CURVE('',#7102,#7101,#5923,.T.);
#8976=EDGE_CURVE('',#7103,#7102,#1841,.T.);
#8977=EDGE_CURVE('',#7103,#7104,#5924,.T.);
#8978=EDGE_CURVE('',#7104,#7105,#1842,.T.);
#8979=EDGE_CURVE('',#7105,#7052,#5925,.T.);
#8980=EDGE_CURVE('',#7106,#7023,#5926,.T.);
#8981=EDGE_CURVE('',#7107,#7022,#5927,.T.);
#8982=EDGE_CURVE('',#7106,#7107,#1843,.T.);
#8983=EDGE_CURVE('',#7108,#7108,#5928,.T.);
#8984=EDGE_CURVE('',#7108,#7109,#1844,.T.);
#8985=EDGE_CURVE('',#7109,#7109,#5929,.T.);
#8986=EDGE_CURVE('',#7084,#7048,#5930,.T.);
#8987=EDGE_CURVE('',#7083,#7026,#5931,.T.);
#8988=EDGE_CURVE('',#7110,#7027,#5932,.T.);
#8989=EDGE_CURVE('',#7111,#7110,#1845,.T.);
#8990=EDGE_CURVE('',#7111,#7049,#5933,.T.);
#8991=EDGE_CURVE('',#7061,#7036,#1846,.T.);
#8992=EDGE_CURVE('',#7035,#7062,#1847,.T.);
#8993=EDGE_CURVE('',#7055,#7014,#1848,.T.);
#8994=EDGE_CURVE('',#7013,#7056,#1849,.T.);
#8995=EDGE_CURVE('',#7112,#7113,#5934,.T.);
#8996=EDGE_CURVE('',#7114,#7112,#1850,.T.);
#8997=EDGE_CURVE('',#7115,#7114,#5935,.T.);
#8998=EDGE_CURVE('',#7113,#7115,#1851,.T.);
#8999=EDGE_CURVE('',#7037,#7060,#1852,.T.);
#9000=EDGE_CURVE('',#7114,#7059,#1853,.T.);
#9001=EDGE_CURVE('',#7112,#7107,#1854,.T.);
#9002=EDGE_CURVE('',#7116,#7113,#1855,.T.);
#9003=EDGE_CURVE('',#7116,#7117,#5936,.T.);
#9004=EDGE_CURVE('',#7117,#7106,#1856,.T.);
#9005=EDGE_CURVE('',#7015,#7054,#1857,.T.);
#9006=EDGE_CURVE('',#7118,#7105,#1858,.T.);
#9007=EDGE_CURVE('',#7118,#7119,#1859,.T.);
#9008=EDGE_CURVE('',#7119,#7098,#1860,.T.);
#9009=EDGE_CURVE('',#7120,#7116,#1861,.T.);
#9010=EDGE_CURVE('',#7121,#7120,#5937,.T.);
#9011=EDGE_CURVE('',#7117,#7121,#1862,.T.);
#9012=EDGE_CURVE('',#7057,#7012,#1863,.T.);
#9013=EDGE_CURVE('',#7063,#7034,#1864,.T.);
#9014=EDGE_CURVE('',#7122,#7097,#1865,.T.);
#9015=EDGE_CURVE('',#7122,#7123,#1866,.T.);
#9016=EDGE_CURVE('',#7123,#7100,#1867,.T.);
#9017=EDGE_CURVE('',#7121,#7058,#1868,.T.);
#9018=EDGE_CURVE('',#7115,#7120,#1869,.T.);
#9019=EDGE_CURVE('',#7102,#7025,#1870,.T.);
#9020=EDGE_CURVE('',#7024,#7103,#1871,.T.);
#9021=EDGE_CURVE('',#7124,#7122,#5938,.T.);
#9022=EDGE_CURVE('',#7125,#7124,#1872,.T.);
#9023=EDGE_CURVE('',#7123,#7125,#5939,.T.);
#9024=EDGE_CURVE('',#7126,#7124,#1873,.T.);
#9025=EDGE_CURVE('',#7126,#7127,#1874,.T.);
#9026=EDGE_CURVE('',#7125,#7127,#1875,.T.);
#9027=EDGE_CURVE('',#7127,#7118,#5940,.T.);
#9028=EDGE_CURVE('',#7104,#7128,#1876,.T.);
#9029=EDGE_CURVE('',#7128,#7129,#1877,.T.);
#9030=EDGE_CURVE('',#7101,#7129,#1878,.T.);
#9031=EDGE_CURVE('',#7130,#7128,#1879,.T.);
#9032=EDGE_CURVE('',#7131,#7130,#1880,.T.);
#9033=EDGE_CURVE('',#7129,#7131,#1881,.T.);
#9034=EDGE_CURVE('',#7099,#7130,#1882,.T.);
#9035=EDGE_CURVE('',#7119,#7126,#5941,.T.);
#9036=EDGE_CURVE('',#7096,#7131,#1883,.T.);
#9037=EDGE_CURVE('',#7092,#7111,#1884,.T.);
#9038=EDGE_CURVE('',#7110,#7093,#1885,.T.);
#9039=EDGE_CURVE('',#7132,#7133,#5942,.T.);
#9040=EDGE_CURVE('',#7134,#7132,#1886,.T.);
#9041=EDGE_CURVE('',#7135,#7134,#5943,.T.);
#9042=EDGE_CURVE('',#7133,#7135,#1887,.T.);
#9043=EDGE_CURVE('',#7136,#7132,#1888,.T.);
#9044=EDGE_CURVE('',#7136,#7137,#1889,.T.);
#9045=EDGE_CURVE('',#7134,#7137,#1890,.T.);
#9046=EDGE_CURVE('',#7137,#7138,#5944,.T.);
#9047=EDGE_CURVE('',#7138,#7095,#1891,.T.);
#9048=EDGE_CURVE('',#7094,#7139,#1892,.T.);
#9049=EDGE_CURVE('',#7139,#7140,#1893,.T.);
#9050=EDGE_CURVE('',#7091,#7140,#1894,.T.);
#9051=EDGE_CURVE('',#7135,#7090,#1895,.T.);
#9052=EDGE_CURVE('',#7141,#7139,#1896,.T.);
#9053=EDGE_CURVE('',#7142,#7141,#1897,.T.);
#9054=EDGE_CURVE('',#7140,#7142,#1898,.T.);
#9055=EDGE_CURVE('',#7089,#7141,#1899,.T.);
#9056=EDGE_CURVE('',#7143,#7088,#1900,.T.);
#9057=EDGE_CURVE('',#7143,#7136,#5945,.T.);
#9058=EDGE_CURVE('',#7133,#7087,#1901,.T.);
#9059=EDGE_CURVE('',#7086,#7142,#1902,.T.);
#9060=EDGE_CURVE('',#7138,#7143,#1903,.T.);
#9061=EDGE_CURVE('',#7031,#7066,#1904,.T.);
#9062=EDGE_CURVE('',#7075,#7044,#1905,.T.);
#9063=EDGE_CURVE('',#7073,#7046,#1906,.T.);
#9064=EDGE_CURVE('',#7045,#7074,#1907,.T.);
#9065=EDGE_CURVE('',#7067,#7030,#1908,.T.);
#9066=EDGE_CURVE('',#7029,#7068,#1909,.T.);
#9067=EDGE_CURVE('',#7144,#7145,#5946,.T.);
#9068=EDGE_CURVE('',#7146,#7144,#1910,.T.);
#9069=EDGE_CURVE('',#7147,#7146,#5947,.T.);
#9070=EDGE_CURVE('',#7145,#7147,#1911,.T.);
#9071=EDGE_CURVE('',#7047,#7072,#1912,.T.);
#9072=EDGE_CURVE('',#7146,#7071,#1913,.T.);
#9073=EDGE_CURVE('',#7144,#7085,#1914,.T.);
#9074=EDGE_CURVE('',#7148,#7145,#1915,.T.);
#9075=EDGE_CURVE('',#7148,#7149,#5948,.T.);
#9076=EDGE_CURVE('',#7149,#7082,#1916,.T.);
#9077=EDGE_CURVE('',#7150,#7148,#1917,.T.);
#9078=EDGE_CURVE('',#7151,#7150,#5949,.T.);
#9079=EDGE_CURVE('',#7149,#7151,#1918,.T.);
#9080=EDGE_CURVE('',#7069,#7028,#1919,.T.);
#9081=EDGE_CURVE('',#7151,#7070,#1920,.T.);
#9082=EDGE_CURVE('',#7147,#7150,#1921,.T.);
#9083=EDGE_CURVE('',#7152,#7153,#1922,.T.);
#9084=EDGE_CURVE('',#7154,#7153,#1923,.T.);
#9085=EDGE_CURVE('',#7155,#7154,#1924,.T.);
#9086=EDGE_CURVE('',#7155,#7152,#1925,.T.);
#9087=EDGE_CURVE('',#7153,#7156,#1926,.T.);
#9088=EDGE_CURVE('',#7157,#7156,#1927,.T.);
#9089=EDGE_CURVE('',#7154,#7157,#1928,.T.);
#9090=EDGE_CURVE('',#7158,#7159,#1929,.T.);
#9091=EDGE_CURVE('',#7159,#7160,#1930,.T.);
#9092=EDGE_CURVE('',#7161,#7160,#1931,.T.);
#9093=EDGE_CURVE('',#7161,#7158,#1932,.T.);
#9094=EDGE_CURVE('',#7162,#7161,#5950,.T.);
#9095=EDGE_CURVE('',#7163,#7162,#1933,.T.);
#9096=EDGE_CURVE('',#7158,#7163,#5951,.T.);
#9097=EDGE_CURVE('',#7164,#7162,#1934,.T.);
#9098=EDGE_CURVE('',#7164,#7165,#1935,.T.);
#9099=EDGE_CURVE('',#7165,#7163,#1936,.T.);
#9100=EDGE_CURVE('',#7166,#7164,#5952,.T.);
#9101=EDGE_CURVE('',#7167,#7166,#1937,.T.);
#9102=EDGE_CURVE('',#7165,#7167,#5953,.T.);
#9103=EDGE_CURVE('',#7168,#7167,#1938,.T.);
#9104=EDGE_CURVE('',#7169,#7166,#1939,.T.);
#9105=EDGE_CURVE('',#7169,#7168,#1940,.T.);
#9106=EDGE_CURVE('',#7160,#7170,#5954,.T.);
#9107=EDGE_CURVE('',#7170,#7171,#1941,.T.);
#9108=EDGE_CURVE('',#7171,#7169,#5955,.T.);
#9109=EDGE_CURVE('',#7172,#7171,#1942,.T.);
#9110=EDGE_CURVE('',#7168,#7172,#5956,.T.);
#9111=EDGE_CURVE('',#7173,#7172,#1943,.T.);
#9112=EDGE_CURVE('',#7173,#7159,#5957,.T.);
#9113=EDGE_CURVE('',#7156,#7174,#1944,.T.);
#9114=EDGE_CURVE('',#7174,#7152,#1945,.T.);
#9115=EDGE_CURVE('',#7170,#7173,#1946,.T.);
#9116=EDGE_CURVE('',#7175,#7174,#1947,.T.);
#9117=EDGE_CURVE('',#7157,#7175,#1948,.T.);
#9118=EDGE_CURVE('',#7175,#7155,#1949,.T.);
#12327=ORIENTED_EDGE('',*,*,#8870,.F.);
#12328=ORIENTED_EDGE('',*,*,#8871,.T.);
#12329=ORIENTED_EDGE('',*,*,#8872,.T.);
#12330=ORIENTED_EDGE('',*,*,#8873,.F.);
#12331=ORIENTED_EDGE('',*,*,#8874,.T.);
#12332=ORIENTED_EDGE('',*,*,#8875,.F.);
#12333=ORIENTED_EDGE('',*,*,#8876,.T.);
#12334=ORIENTED_EDGE('',*,*,#8877,.F.);
#12335=ORIENTED_EDGE('',*,*,#8876,.F.);
#12336=ORIENTED_EDGE('',*,*,#8878,.F.);
#12337=ORIENTED_EDGE('',*,*,#8879,.T.);
#12338=ORIENTED_EDGE('',*,*,#8880,.F.);
#12339=ORIENTED_EDGE('',*,*,#8881,.T.);
#12340=ORIENTED_EDGE('',*,*,#8882,.F.);
#12341=ORIENTED_EDGE('',*,*,#8883,.F.);
#12342=ORIENTED_EDGE('',*,*,#8884,.T.);
#12343=ORIENTED_EDGE('',*,*,#8870,.T.);
#12344=ORIENTED_EDGE('',*,*,#8885,.F.);
#12345=ORIENTED_EDGE('',*,*,#8886,.F.);
#12346=ORIENTED_EDGE('',*,*,#8887,.T.);
#12347=ORIENTED_EDGE('',*,*,#8888,.F.);
#12348=ORIENTED_EDGE('',*,*,#8889,.T.);
#12349=ORIENTED_EDGE('',*,*,#8890,.T.);
#12350=ORIENTED_EDGE('',*,*,#8891,.F.);
#12351=ORIENTED_EDGE('',*,*,#8892,.T.);
#12352=ORIENTED_EDGE('',*,*,#8893,.F.);
#12353=ORIENTED_EDGE('',*,*,#8894,.T.);
#12354=ORIENTED_EDGE('',*,*,#8895,.T.);
#12355=ORIENTED_EDGE('',*,*,#8896,.T.);
#12356=ORIENTED_EDGE('',*,*,#8897,.T.);
#12357=ORIENTED_EDGE('',*,*,#8898,.T.);
#12358=ORIENTED_EDGE('',*,*,#8899,.F.);
#12359=ORIENTED_EDGE('',*,*,#8881,.F.);
#12360=ORIENTED_EDGE('',*,*,#8900,.T.);
#12361=ORIENTED_EDGE('',*,*,#8901,.T.);
#12362=ORIENTED_EDGE('',*,*,#8902,.T.);
#12363=ORIENTED_EDGE('',*,*,#8894,.F.);
#12364=ORIENTED_EDGE('',*,*,#8903,.F.);
#12365=ORIENTED_EDGE('',*,*,#8904,.T.);
#12366=ORIENTED_EDGE('',*,*,#8905,.F.);
#12367=ORIENTED_EDGE('',*,*,#8906,.F.);
#12368=ORIENTED_EDGE('',*,*,#8907,.T.);
#12369=ORIENTED_EDGE('',*,*,#8908,.T.);
#12370=ORIENTED_EDGE('',*,*,#8909,.T.);
#12371=ORIENTED_EDGE('',*,*,#8910,.T.);
#12372=ORIENTED_EDGE('',*,*,#8911,.T.);
#12373=ORIENTED_EDGE('',*,*,#8912,.F.);
#12374=ORIENTED_EDGE('',*,*,#8913,.F.);
#12375=ORIENTED_EDGE('',*,*,#8914,.T.);
#12376=ORIENTED_EDGE('',*,*,#8915,.T.);
#12377=ORIENTED_EDGE('',*,*,#8916,.T.);
#12378=ORIENTED_EDGE('',*,*,#8907,.F.);
#12379=ORIENTED_EDGE('',*,*,#8917,.F.);
#12380=ORIENTED_EDGE('',*,*,#8918,.T.);
#12381=ORIENTED_EDGE('',*,*,#8919,.T.);
#12382=ORIENTED_EDGE('',*,*,#8920,.F.);
#12383=ORIENTED_EDGE('',*,*,#8921,.T.);
#12384=ORIENTED_EDGE('',*,*,#8922,.F.);
#12385=ORIENTED_EDGE('',*,*,#8923,.F.);
#12386=ORIENTED_EDGE('',*,*,#8924,.T.);
#12387=ORIENTED_EDGE('',*,*,#8925,.T.);
#12388=ORIENTED_EDGE('',*,*,#8926,.T.);
#12389=ORIENTED_EDGE('',*,*,#8927,.T.);
#12390=ORIENTED_EDGE('',*,*,#8928,.F.);
#12391=ORIENTED_EDGE('',*,*,#8929,.F.);
#12392=ORIENTED_EDGE('',*,*,#8930,.T.);
#12393=ORIENTED_EDGE('',*,*,#8931,.T.);
#12394=ORIENTED_EDGE('',*,*,#8932,.F.);
#12395=ORIENTED_EDGE('',*,*,#8933,.T.);
#12396=ORIENTED_EDGE('',*,*,#8934,.F.);
#12397=ORIENTED_EDGE('',*,*,#8935,.F.);
#12398=ORIENTED_EDGE('',*,*,#8936,.T.);
#12399=ORIENTED_EDGE('',*,*,#8937,.T.);
#12400=ORIENTED_EDGE('',*,*,#8938,.T.);
#12401=ORIENTED_EDGE('',*,*,#8939,.T.);
#12402=ORIENTED_EDGE('',*,*,#8940,.F.);
#12403=ORIENTED_EDGE('',*,*,#8941,.F.);
#12404=ORIENTED_EDGE('',*,*,#8942,.T.);
#12405=ORIENTED_EDGE('',*,*,#8943,.T.);
#12406=ORIENTED_EDGE('',*,*,#8942,.F.);
#12407=ORIENTED_EDGE('',*,*,#8944,.T.);
#12408=ORIENTED_EDGE('',*,*,#8945,.T.);
#12409=ORIENTED_EDGE('',*,*,#8946,.T.);
#12410=ORIENTED_EDGE('',*,*,#8945,.F.);
#12411=ORIENTED_EDGE('',*,*,#8947,.F.);
#12412=ORIENTED_EDGE('',*,*,#8948,.T.);
#12413=ORIENTED_EDGE('',*,*,#8949,.T.);
#12414=ORIENTED_EDGE('',*,*,#8948,.F.);
#12415=ORIENTED_EDGE('',*,*,#8950,.T.);
#12416=ORIENTED_EDGE('',*,*,#8951,.T.);
#12417=ORIENTED_EDGE('',*,*,#8952,.F.);
#12418=ORIENTED_EDGE('',*,*,#8953,.F.);
#12419=ORIENTED_EDGE('',*,*,#8954,.T.);
#12420=ORIENTED_EDGE('',*,*,#8955,.T.);
#12421=ORIENTED_EDGE('',*,*,#8956,.T.);
#12422=ORIENTED_EDGE('',*,*,#8915,.F.);
#12423=ORIENTED_EDGE('',*,*,#8957,.F.);
#12424=ORIENTED_EDGE('',*,*,#8958,.T.);
#12425=ORIENTED_EDGE('',*,*,#8959,.F.);
#12426=ORIENTED_EDGE('',*,*,#8904,.F.);
#12427=ORIENTED_EDGE('',*,*,#8929,.T.);
#12428=ORIENTED_EDGE('',*,*,#8960,.F.);
#12429=ORIENTED_EDGE('',*,*,#8961,.T.);
#12430=ORIENTED_EDGE('',*,*,#8962,.F.);
#12431=ORIENTED_EDGE('',*,*,#8963,.F.);
#12432=ORIENTED_EDGE('',*,*,#8964,.T.);
#12433=ORIENTED_EDGE('',*,*,#8965,.T.);
#12434=ORIENTED_EDGE('',*,*,#8966,.T.);
#12435=ORIENTED_EDGE('',*,*,#8967,.T.);
#12436=ORIENTED_EDGE('',*,*,#8968,.T.);
#12437=ORIENTED_EDGE('',*,*,#8969,.T.);
#12438=ORIENTED_EDGE('',*,*,#8901,.F.);
#12439=ORIENTED_EDGE('',*,*,#8970,.F.);
#12440=ORIENTED_EDGE('',*,*,#8971,.T.);
#12441=ORIENTED_EDGE('',*,*,#8972,.F.);
#12442=ORIENTED_EDGE('',*,*,#8879,.F.);
#12443=ORIENTED_EDGE('',*,*,#8917,.T.);
#12444=ORIENTED_EDGE('',*,*,#8973,.F.);
#12445=ORIENTED_EDGE('',*,*,#8974,.T.);
#12446=ORIENTED_EDGE('',*,*,#8975,.F.);
#12447=ORIENTED_EDGE('',*,*,#8976,.F.);
#12448=ORIENTED_EDGE('',*,*,#8977,.T.);
#12449=ORIENTED_EDGE('',*,*,#8978,.T.);
#12450=ORIENTED_EDGE('',*,*,#8979,.T.);
#12451=ORIENTED_EDGE('',*,*,#8980,.T.);
#12452=ORIENTED_EDGE('',*,*,#8883,.T.);
#12453=ORIENTED_EDGE('',*,*,#8981,.F.);
#12454=ORIENTED_EDGE('',*,*,#8982,.F.);
#12455=ORIENTED_EDGE('',*,*,#8983,.T.);
#12456=ORIENTED_EDGE('',*,*,#8984,.T.);
#12457=ORIENTED_EDGE('',*,*,#8985,.F.);
#12458=ORIENTED_EDGE('',*,*,#8984,.F.);
#12459=ORIENTED_EDGE('',*,*,#8913,.T.);
#12460=ORIENTED_EDGE('',*,*,#8986,.F.);
#12461=ORIENTED_EDGE('',*,*,#8951,.F.);
#12462=ORIENTED_EDGE('',*,*,#8987,.T.);
#12463=ORIENTED_EDGE('',*,*,#8888,.T.);
#12464=ORIENTED_EDGE('',*,*,#8988,.F.);
#12465=ORIENTED_EDGE('',*,*,#8989,.F.);
#12466=ORIENTED_EDGE('',*,*,#8990,.T.);
#12467=ORIENTED_EDGE('',*,*,#8877,.T.);
#12468=ORIENTED_EDGE('',*,*,#8983,.F.);
#12469=ORIENTED_EDGE('',*,*,#8926,.F.);
#12470=ORIENTED_EDGE('',*,*,#8991,.T.);
#12471=ORIENTED_EDGE('',*,*,#8897,.F.);
#12472=ORIENTED_EDGE('',*,*,#8992,.T.);
#12473=ORIENTED_EDGE('',*,*,#8920,.T.);
#12474=ORIENTED_EDGE('',*,*,#8993,.T.);
#12475=ORIENTED_EDGE('',*,*,#8873,.T.);
#12476=ORIENTED_EDGE('',*,*,#8994,.T.);
#12477=ORIENTED_EDGE('',*,*,#8995,.F.);
#12478=ORIENTED_EDGE('',*,*,#8996,.F.);
#12479=ORIENTED_EDGE('',*,*,#8997,.F.);
#12480=ORIENTED_EDGE('',*,*,#8998,.F.);
#12481=ORIENTED_EDGE('',*,*,#8882,.T.);
#12482=ORIENTED_EDGE('',*,*,#8899,.T.);
#12483=ORIENTED_EDGE('',*,*,#8999,.T.);
#12484=ORIENTED_EDGE('',*,*,#8924,.F.);
#12485=ORIENTED_EDGE('',*,*,#9000,.F.);
#12486=ORIENTED_EDGE('',*,*,#8996,.T.);
#12487=ORIENTED_EDGE('',*,*,#9001,.T.);
#12488=ORIENTED_EDGE('',*,*,#8981,.T.);
#12489=ORIENTED_EDGE('',*,*,#9002,.F.);
#12490=ORIENTED_EDGE('',*,*,#9003,.T.);
#12491=ORIENTED_EDGE('',*,*,#9004,.T.);
#12492=ORIENTED_EDGE('',*,*,#8982,.T.);
#12493=ORIENTED_EDGE('',*,*,#9001,.F.);
#12494=ORIENTED_EDGE('',*,*,#8995,.T.);
#12495=ORIENTED_EDGE('',*,*,#8898,.F.);
#12496=ORIENTED_EDGE('',*,*,#8991,.F.);
#12497=ORIENTED_EDGE('',*,*,#8925,.F.);
#12498=ORIENTED_EDGE('',*,*,#8999,.F.);
#12499=ORIENTED_EDGE('',*,*,#8878,.T.);
#12500=ORIENTED_EDGE('',*,*,#8875,.T.);
#12501=ORIENTED_EDGE('',*,*,#9005,.T.);
#12502=ORIENTED_EDGE('',*,*,#8918,.F.);
#12503=ORIENTED_EDGE('',*,*,#8979,.F.);
#12504=ORIENTED_EDGE('',*,*,#9006,.F.);
#12505=ORIENTED_EDGE('',*,*,#9007,.T.);
#12506=ORIENTED_EDGE('',*,*,#9008,.T.);
#12507=ORIENTED_EDGE('',*,*,#8970,.T.);
#12508=ORIENTED_EDGE('',*,*,#9003,.F.);
#12509=ORIENTED_EDGE('',*,*,#9009,.F.);
#12510=ORIENTED_EDGE('',*,*,#9010,.F.);
#12511=ORIENTED_EDGE('',*,*,#9011,.F.);
#12512=ORIENTED_EDGE('',*,*,#8872,.F.);
#12513=ORIENTED_EDGE('',*,*,#9012,.F.);
#12514=ORIENTED_EDGE('',*,*,#8921,.F.);
#12515=ORIENTED_EDGE('',*,*,#8994,.F.);
#12516=ORIENTED_EDGE('',*,*,#8927,.F.);
#12517=ORIENTED_EDGE('',*,*,#8992,.F.);
#12518=ORIENTED_EDGE('',*,*,#8896,.F.);
#12519=ORIENTED_EDGE('',*,*,#9013,.F.);
#12520=ORIENTED_EDGE('',*,*,#8973,.T.);
#12521=ORIENTED_EDGE('',*,*,#8928,.T.);
#12522=ORIENTED_EDGE('',*,*,#9013,.T.);
#12523=ORIENTED_EDGE('',*,*,#8895,.F.);
#12524=ORIENTED_EDGE('',*,*,#8902,.F.);
#12525=ORIENTED_EDGE('',*,*,#8969,.F.);
#12526=ORIENTED_EDGE('',*,*,#9014,.F.);
#12527=ORIENTED_EDGE('',*,*,#9015,.T.);
#12528=ORIENTED_EDGE('',*,*,#9016,.T.);
#12529=ORIENTED_EDGE('',*,*,#9017,.F.);
#12530=ORIENTED_EDGE('',*,*,#9010,.T.);
#12531=ORIENTED_EDGE('',*,*,#9018,.F.);
#12532=ORIENTED_EDGE('',*,*,#8997,.T.);
#12533=ORIENTED_EDGE('',*,*,#9000,.T.);
#12534=ORIENTED_EDGE('',*,*,#8923,.T.);
#12535=ORIENTED_EDGE('',*,*,#8922,.T.);
#12536=ORIENTED_EDGE('',*,*,#9012,.T.);
#12537=ORIENTED_EDGE('',*,*,#8871,.F.);
#12538=ORIENTED_EDGE('',*,*,#8884,.F.);
#12539=ORIENTED_EDGE('',*,*,#8980,.F.);
#12540=ORIENTED_EDGE('',*,*,#9004,.F.);
#12541=ORIENTED_EDGE('',*,*,#9011,.T.);
#12542=ORIENTED_EDGE('',*,*,#9017,.T.);
#12543=ORIENTED_EDGE('',*,*,#8919,.F.);
#12544=ORIENTED_EDGE('',*,*,#9005,.F.);
#12545=ORIENTED_EDGE('',*,*,#8874,.F.);
#12546=ORIENTED_EDGE('',*,*,#8993,.F.);
#12547=ORIENTED_EDGE('',*,*,#9018,.T.);
#12548=ORIENTED_EDGE('',*,*,#9009,.T.);
#12549=ORIENTED_EDGE('',*,*,#9002,.T.);
#12550=ORIENTED_EDGE('',*,*,#8998,.T.);
#12551=ORIENTED_EDGE('',*,*,#8976,.T.);
#12552=ORIENTED_EDGE('',*,*,#9019,.T.);
#12553=ORIENTED_EDGE('',*,*,#8886,.T.);
#12554=ORIENTED_EDGE('',*,*,#9020,.T.);
#12555=ORIENTED_EDGE('',*,*,#9021,.F.);
#12556=ORIENTED_EDGE('',*,*,#9022,.F.);
#12557=ORIENTED_EDGE('',*,*,#9023,.F.);
#12558=ORIENTED_EDGE('',*,*,#9015,.F.);
#12559=ORIENTED_EDGE('',*,*,#9024,.F.);
#12560=ORIENTED_EDGE('',*,*,#9025,.T.);
#12561=ORIENTED_EDGE('',*,*,#9026,.F.);
#12562=ORIENTED_EDGE('',*,*,#9022,.T.);
#12563=ORIENTED_EDGE('',*,*,#9026,.T.);
#12564=ORIENTED_EDGE('',*,*,#9027,.T.);
#12565=ORIENTED_EDGE('',*,*,#9006,.T.);
#12566=ORIENTED_EDGE('',*,*,#8978,.F.);
#12567=ORIENTED_EDGE('',*,*,#9028,.T.);
#12568=ORIENTED_EDGE('',*,*,#9029,.T.);
#12569=ORIENTED_EDGE('',*,*,#9030,.F.);
#12570=ORIENTED_EDGE('',*,*,#8974,.F.);
#12571=ORIENTED_EDGE('',*,*,#9016,.F.);
#12572=ORIENTED_EDGE('',*,*,#9023,.T.);
#12573=ORIENTED_EDGE('',*,*,#9029,.F.);
#12574=ORIENTED_EDGE('',*,*,#9031,.F.);
#12575=ORIENTED_EDGE('',*,*,#9032,.F.);
#12576=ORIENTED_EDGE('',*,*,#9033,.F.);
#12577=ORIENTED_EDGE('',*,*,#8977,.F.);
#12578=ORIENTED_EDGE('',*,*,#9020,.F.);
#12579=ORIENTED_EDGE('',*,*,#8885,.T.);
#12580=ORIENTED_EDGE('',*,*,#8880,.T.);
#12581=ORIENTED_EDGE('',*,*,#8972,.T.);
#12582=ORIENTED_EDGE('',*,*,#9034,.T.);
#12583=ORIENTED_EDGE('',*,*,#9031,.T.);
#12584=ORIENTED_EDGE('',*,*,#9028,.F.);
#12585=ORIENTED_EDGE('',*,*,#9008,.F.);
#12586=ORIENTED_EDGE('',*,*,#9035,.T.);
#12587=ORIENTED_EDGE('',*,*,#9024,.T.);
#12588=ORIENTED_EDGE('',*,*,#9021,.T.);
#12589=ORIENTED_EDGE('',*,*,#9014,.T.);
#12590=ORIENTED_EDGE('',*,*,#8968,.F.);
#12591=ORIENTED_EDGE('',*,*,#9036,.T.);
#12592=ORIENTED_EDGE('',*,*,#9032,.T.);
#12593=ORIENTED_EDGE('',*,*,#9034,.F.);
#12594=ORIENTED_EDGE('',*,*,#8971,.F.);
#12595=ORIENTED_EDGE('',*,*,#8887,.F.);
#12596=ORIENTED_EDGE('',*,*,#9019,.F.);
#12597=ORIENTED_EDGE('',*,*,#8975,.T.);
#12598=ORIENTED_EDGE('',*,*,#9030,.T.);
#12599=ORIENTED_EDGE('',*,*,#9033,.T.);
#12600=ORIENTED_EDGE('',*,*,#9036,.F.);
#12601=ORIENTED_EDGE('',*,*,#8967,.F.);
#12602=ORIENTED_EDGE('',*,*,#8900,.F.);
#12603=ORIENTED_EDGE('',*,*,#9027,.F.);
#12604=ORIENTED_EDGE('',*,*,#9025,.F.);
#12605=ORIENTED_EDGE('',*,*,#9035,.F.);
#12606=ORIENTED_EDGE('',*,*,#9007,.F.);
#12607=ORIENTED_EDGE('',*,*,#8963,.T.);
#12608=ORIENTED_EDGE('',*,*,#9037,.T.);
#12609=ORIENTED_EDGE('',*,*,#8989,.T.);
#12610=ORIENTED_EDGE('',*,*,#9038,.T.);
#12611=ORIENTED_EDGE('',*,*,#9039,.F.);
#12612=ORIENTED_EDGE('',*,*,#9040,.F.);
#12613=ORIENTED_EDGE('',*,*,#9041,.F.);
#12614=ORIENTED_EDGE('',*,*,#9042,.F.);
#12615=ORIENTED_EDGE('',*,*,#9043,.F.);
#12616=ORIENTED_EDGE('',*,*,#9044,.T.);
#12617=ORIENTED_EDGE('',*,*,#9045,.F.);
#12618=ORIENTED_EDGE('',*,*,#9040,.T.);
#12619=ORIENTED_EDGE('',*,*,#9045,.T.);
#12620=ORIENTED_EDGE('',*,*,#9046,.T.);
#12621=ORIENTED_EDGE('',*,*,#9047,.T.);
#12622=ORIENTED_EDGE('',*,*,#8965,.F.);
#12623=ORIENTED_EDGE('',*,*,#9048,.T.);
#12624=ORIENTED_EDGE('',*,*,#9049,.T.);
#12625=ORIENTED_EDGE('',*,*,#9050,.F.);
#12626=ORIENTED_EDGE('',*,*,#8961,.F.);
#12627=ORIENTED_EDGE('',*,*,#9051,.F.);
#12628=ORIENTED_EDGE('',*,*,#9041,.T.);
#12629=ORIENTED_EDGE('',*,*,#9049,.F.);
#12630=ORIENTED_EDGE('',*,*,#9052,.F.);
#12631=ORIENTED_EDGE('',*,*,#9053,.F.);
#12632=ORIENTED_EDGE('',*,*,#9054,.F.);
#12633=ORIENTED_EDGE('',*,*,#8964,.F.);
#12634=ORIENTED_EDGE('',*,*,#9038,.F.);
#12635=ORIENTED_EDGE('',*,*,#8988,.T.);
#12636=ORIENTED_EDGE('',*,*,#8905,.T.);
#12637=ORIENTED_EDGE('',*,*,#8959,.T.);
#12638=ORIENTED_EDGE('',*,*,#9055,.T.);
#12639=ORIENTED_EDGE('',*,*,#9052,.T.);
#12640=ORIENTED_EDGE('',*,*,#9048,.F.);
#12641=ORIENTED_EDGE('',*,*,#9056,.F.);
#12642=ORIENTED_EDGE('',*,*,#9057,.T.);
#12643=ORIENTED_EDGE('',*,*,#9043,.T.);
#12644=ORIENTED_EDGE('',*,*,#9039,.T.);
#12645=ORIENTED_EDGE('',*,*,#9058,.T.);
#12646=ORIENTED_EDGE('',*,*,#8955,.F.);
#12647=ORIENTED_EDGE('',*,*,#9059,.T.);
#12648=ORIENTED_EDGE('',*,*,#9053,.T.);
#12649=ORIENTED_EDGE('',*,*,#9055,.F.);
#12650=ORIENTED_EDGE('',*,*,#8958,.F.);
#12651=ORIENTED_EDGE('',*,*,#9047,.F.);
#12652=ORIENTED_EDGE('',*,*,#9060,.T.);
#12653=ORIENTED_EDGE('',*,*,#9056,.T.);
#12654=ORIENTED_EDGE('',*,*,#8957,.T.);
#12655=ORIENTED_EDGE('',*,*,#8903,.T.);
#12656=ORIENTED_EDGE('',*,*,#8893,.T.);
#12657=ORIENTED_EDGE('',*,*,#9061,.T.);
#12658=ORIENTED_EDGE('',*,*,#8930,.F.);
#12659=ORIENTED_EDGE('',*,*,#8966,.F.);
#12660=ORIENTED_EDGE('',*,*,#9058,.F.);
#12661=ORIENTED_EDGE('',*,*,#9042,.T.);
#12662=ORIENTED_EDGE('',*,*,#9051,.T.);
#12663=ORIENTED_EDGE('',*,*,#8960,.T.);
#12664=ORIENTED_EDGE('',*,*,#8940,.T.);
#12665=ORIENTED_EDGE('',*,*,#9062,.T.);
#12666=ORIENTED_EDGE('',*,*,#8908,.F.);
#12667=ORIENTED_EDGE('',*,*,#8916,.F.);
#12668=ORIENTED_EDGE('',*,*,#8956,.F.);
#12669=ORIENTED_EDGE('',*,*,#8990,.F.);
#12670=ORIENTED_EDGE('',*,*,#9037,.F.);
#12671=ORIENTED_EDGE('',*,*,#8962,.T.);
#12672=ORIENTED_EDGE('',*,*,#9050,.T.);
#12673=ORIENTED_EDGE('',*,*,#9054,.T.);
#12674=ORIENTED_EDGE('',*,*,#9059,.F.);
#12675=ORIENTED_EDGE('',*,*,#8954,.F.);
#12676=ORIENTED_EDGE('',*,*,#8914,.F.);
#12677=ORIENTED_EDGE('',*,*,#9046,.F.);
#12678=ORIENTED_EDGE('',*,*,#9044,.F.);
#12679=ORIENTED_EDGE('',*,*,#9057,.F.);
#12680=ORIENTED_EDGE('',*,*,#9060,.F.);
#12681=ORIENTED_EDGE('',*,*,#8938,.F.);
#12682=ORIENTED_EDGE('',*,*,#9063,.T.);
#12683=ORIENTED_EDGE('',*,*,#8910,.F.);
#12684=ORIENTED_EDGE('',*,*,#9064,.T.);
#12685=ORIENTED_EDGE('',*,*,#8932,.T.);
#12686=ORIENTED_EDGE('',*,*,#9065,.T.);
#12687=ORIENTED_EDGE('',*,*,#8891,.T.);
#12688=ORIENTED_EDGE('',*,*,#9066,.T.);
#12689=ORIENTED_EDGE('',*,*,#9067,.F.);
#12690=ORIENTED_EDGE('',*,*,#9068,.F.);
#12691=ORIENTED_EDGE('',*,*,#9069,.F.);
#12692=ORIENTED_EDGE('',*,*,#9070,.F.);
#12693=ORIENTED_EDGE('',*,*,#8986,.T.);
#12694=ORIENTED_EDGE('',*,*,#8912,.T.);
#12695=ORIENTED_EDGE('',*,*,#9071,.T.);
#12696=ORIENTED_EDGE('',*,*,#8936,.F.);
#12697=ORIENTED_EDGE('',*,*,#9072,.F.);
#12698=ORIENTED_EDGE('',*,*,#9068,.T.);
#12699=ORIENTED_EDGE('',*,*,#9073,.T.);
#12700=ORIENTED_EDGE('',*,*,#8952,.T.);
#12701=ORIENTED_EDGE('',*,*,#9074,.F.);
#12702=ORIENTED_EDGE('',*,*,#9075,.T.);
#12703=ORIENTED_EDGE('',*,*,#9076,.T.);
#12704=ORIENTED_EDGE('',*,*,#8953,.T.);
#12705=ORIENTED_EDGE('',*,*,#9073,.F.);
#12706=ORIENTED_EDGE('',*,*,#9067,.T.);
#12707=ORIENTED_EDGE('',*,*,#8911,.F.);
#12708=ORIENTED_EDGE('',*,*,#9063,.F.);
#12709=ORIENTED_EDGE('',*,*,#8937,.F.);
#12710=ORIENTED_EDGE('',*,*,#9071,.F.);
#12711=ORIENTED_EDGE('',*,*,#9075,.F.);
#12712=ORIENTED_EDGE('',*,*,#9077,.F.);
#12713=ORIENTED_EDGE('',*,*,#9078,.F.);
#12714=ORIENTED_EDGE('',*,*,#9079,.F.);
#12715=ORIENTED_EDGE('',*,*,#8890,.F.);
#12716=ORIENTED_EDGE('',*,*,#9080,.F.);
#12717=ORIENTED_EDGE('',*,*,#8933,.F.);
#12718=ORIENTED_EDGE('',*,*,#9066,.F.);
#12719=ORIENTED_EDGE('',*,*,#8939,.F.);
#12720=ORIENTED_EDGE('',*,*,#9064,.F.);
#12721=ORIENTED_EDGE('',*,*,#8909,.F.);
#12722=ORIENTED_EDGE('',*,*,#9062,.F.);
#12723=ORIENTED_EDGE('',*,*,#9081,.F.);
#12724=ORIENTED_EDGE('',*,*,#9078,.T.);
#12725=ORIENTED_EDGE('',*,*,#9082,.F.);
#12726=ORIENTED_EDGE('',*,*,#9069,.T.);
#12727=ORIENTED_EDGE('',*,*,#9072,.T.);
#12728=ORIENTED_EDGE('',*,*,#8935,.T.);
#12729=ORIENTED_EDGE('',*,*,#8934,.T.);
#12730=ORIENTED_EDGE('',*,*,#9080,.T.);
#12731=ORIENTED_EDGE('',*,*,#8889,.F.);
#12732=ORIENTED_EDGE('',*,*,#8987,.F.);
#12733=ORIENTED_EDGE('',*,*,#8950,.F.);
#12734=ORIENTED_EDGE('',*,*,#9076,.F.);
#12735=ORIENTED_EDGE('',*,*,#9079,.T.);
#12736=ORIENTED_EDGE('',*,*,#9081,.T.);
#12737=ORIENTED_EDGE('',*,*,#8931,.F.);
#12738=ORIENTED_EDGE('',*,*,#9061,.F.);
#12739=ORIENTED_EDGE('',*,*,#8892,.F.);
#12740=ORIENTED_EDGE('',*,*,#9065,.F.);
#12741=ORIENTED_EDGE('',*,*,#9082,.T.);
#12742=ORIENTED_EDGE('',*,*,#9077,.T.);
#12743=ORIENTED_EDGE('',*,*,#9074,.T.);
#12744=ORIENTED_EDGE('',*,*,#9070,.T.);
#12745=ORIENTED_EDGE('',*,*,#8949,.F.);
#12746=ORIENTED_EDGE('',*,*,#8944,.F.);
#12747=ORIENTED_EDGE('',*,*,#8947,.T.);
#12748=ORIENTED_EDGE('',*,*,#8985,.T.);
#12749=ORIENTED_EDGE('',*,*,#8946,.F.);
#12750=ORIENTED_EDGE('',*,*,#8943,.F.);
#12751=ORIENTED_EDGE('',*,*,#9083,.T.);
#12752=ORIENTED_EDGE('',*,*,#9084,.F.);
#12753=ORIENTED_EDGE('',*,*,#9085,.F.);
#12754=ORIENTED_EDGE('',*,*,#9086,.T.);
#12755=ORIENTED_EDGE('',*,*,#9087,.T.);
#12756=ORIENTED_EDGE('',*,*,#9088,.F.);
#12757=ORIENTED_EDGE('',*,*,#9089,.F.);
#12758=ORIENTED_EDGE('',*,*,#9084,.T.);
#12759=ORIENTED_EDGE('',*,*,#9090,.T.);
#12760=ORIENTED_EDGE('',*,*,#9091,.T.);
#12761=ORIENTED_EDGE('',*,*,#9092,.F.);
#12762=ORIENTED_EDGE('',*,*,#9093,.T.);
#12763=ORIENTED_EDGE('',*,*,#9094,.F.);
#12764=ORIENTED_EDGE('',*,*,#9095,.F.);
#12765=ORIENTED_EDGE('',*,*,#9096,.F.);
#12766=ORIENTED_EDGE('',*,*,#9093,.F.);
#12767=ORIENTED_EDGE('',*,*,#9097,.F.);
#12768=ORIENTED_EDGE('',*,*,#9098,.T.);
#12769=ORIENTED_EDGE('',*,*,#9099,.T.);
#12770=ORIENTED_EDGE('',*,*,#9095,.T.);
#12771=ORIENTED_EDGE('',*,*,#9100,.F.);
#12772=ORIENTED_EDGE('',*,*,#9101,.F.);
#12773=ORIENTED_EDGE('',*,*,#9102,.F.);
#12774=ORIENTED_EDGE('',*,*,#9098,.F.);
#12775=ORIENTED_EDGE('',*,*,#9103,.T.);
#12776=ORIENTED_EDGE('',*,*,#9101,.T.);
#12777=ORIENTED_EDGE('',*,*,#9104,.F.);
#12778=ORIENTED_EDGE('',*,*,#9105,.T.);
#12779=ORIENTED_EDGE('',*,*,#9092,.T.);
#12780=ORIENTED_EDGE('',*,*,#9106,.T.);
#12781=ORIENTED_EDGE('',*,*,#9107,.T.);
#12782=ORIENTED_EDGE('',*,*,#9108,.T.);
#12783=ORIENTED_EDGE('',*,*,#9104,.T.);
#12784=ORIENTED_EDGE('',*,*,#9100,.T.);
#12785=ORIENTED_EDGE('',*,*,#9097,.T.);
#12786=ORIENTED_EDGE('',*,*,#9094,.T.);
#12787=ORIENTED_EDGE('',*,*,#8941,.T.);
#12788=ORIENTED_EDGE('',*,*,#9108,.F.);
#12789=ORIENTED_EDGE('',*,*,#9109,.F.);
#12790=ORIENTED_EDGE('',*,*,#9110,.F.);
#12791=ORIENTED_EDGE('',*,*,#9105,.F.);
#12792=ORIENTED_EDGE('',*,*,#9111,.F.);
#12793=ORIENTED_EDGE('',*,*,#9112,.T.);
#12794=ORIENTED_EDGE('',*,*,#9090,.F.);
#12795=ORIENTED_EDGE('',*,*,#9096,.T.);
#12796=ORIENTED_EDGE('',*,*,#9099,.F.);
#12797=ORIENTED_EDGE('',*,*,#9102,.T.);
#12798=ORIENTED_EDGE('',*,*,#9103,.F.);
#12799=ORIENTED_EDGE('',*,*,#9110,.T.);
#12800=ORIENTED_EDGE('',*,*,#9113,.F.);
#12801=ORIENTED_EDGE('',*,*,#9087,.F.);
#12802=ORIENTED_EDGE('',*,*,#9083,.F.);
#12803=ORIENTED_EDGE('',*,*,#9114,.F.);
#12804=ORIENTED_EDGE('',*,*,#9107,.F.);
#12805=ORIENTED_EDGE('',*,*,#9115,.T.);
#12806=ORIENTED_EDGE('',*,*,#9111,.T.);
#12807=ORIENTED_EDGE('',*,*,#9109,.T.);
#12808=ORIENTED_EDGE('',*,*,#9113,.T.);
#12809=ORIENTED_EDGE('',*,*,#9116,.F.);
#12810=ORIENTED_EDGE('',*,*,#9117,.F.);
#12811=ORIENTED_EDGE('',*,*,#9088,.T.);
#12812=ORIENTED_EDGE('',*,*,#9117,.T.);
#12813=ORIENTED_EDGE('',*,*,#9118,.T.);
#12814=ORIENTED_EDGE('',*,*,#9085,.T.);
#12815=ORIENTED_EDGE('',*,*,#9089,.T.);
#12816=ORIENTED_EDGE('',*,*,#8906,.T.);
#12817=ORIENTED_EDGE('',*,*,#9114,.T.);
#12818=ORIENTED_EDGE('',*,*,#9086,.F.);
#12819=ORIENTED_EDGE('',*,*,#9118,.F.);
#12820=ORIENTED_EDGE('',*,*,#9116,.T.);
#12821=ORIENTED_EDGE('',*,*,#9106,.F.);
#12822=ORIENTED_EDGE('',*,*,#9091,.F.);
#12823=ORIENTED_EDGE('',*,*,#9112,.F.);
#12824=ORIENTED_EDGE('',*,*,#9115,.F.);
#14821=ADVANCED_FACE('',(#4186),#3547,.T.);
#14822=ADVANCED_FACE('',(#4187),#3548,.T.);
#14823=ADVANCED_FACE('',(#4188),#3549,.T.);
#14824=ADVANCED_FACE('',(#4189),#3550,.T.);
#14825=ADVANCED_FACE('',(#4190),#3551,.T.);
#14826=ADVANCED_FACE('',(#4191),#3552,.T.);
#14827=ADVANCED_FACE('',(#4192),#3553,.F.);
#14828=ADVANCED_FACE('',(#4193),#3554,.T.);
#14829=ADVANCED_FACE('',(#4194),#3555,.F.);
#14830=ADVANCED_FACE('',(#4195),#3556,.T.);
#14831=ADVANCED_FACE('',(#4196),#3557,.T.);
#14832=ADVANCED_FACE('',(#4197),#3558,.T.);
#14833=ADVANCED_FACE('',(#4198),#3559,.T.);
#14834=ADVANCED_FACE('',(#4199),#3560,.T.);
#14835=ADVANCED_FACE('',(#4200),#3561,.T.);
#14836=ADVANCED_FACE('',(#4201),#3562,.T.);
#14837=ADVANCED_FACE('',(#4202),#3563,.T.);
#14838=ADVANCED_FACE('',(#4203),#3564,.F.);
#14839=ADVANCED_FACE('',(#4204),#3565,.T.);
#14840=ADVANCED_FACE('',(#4205,#234),#589,.T.);
#14841=ADVANCED_FACE('',(#4206),#590,.T.);
#14842=ADVANCED_FACE('',(#4207),#591,.F.);
#14843=ADVANCED_FACE('',(#4208),#3566,.T.);
#14844=ADVANCED_FACE('',(#4209),#592,.F.);
#14845=ADVANCED_FACE('',(#4210),#593,.T.);
#14846=ADVANCED_FACE('',(#4211),#3567,.F.);
#14847=ADVANCED_FACE('',(#4212),#594,.T.);
#14848=ADVANCED_FACE('',(#4213),#3568,.T.);
#14849=ADVANCED_FACE('',(#4214),#3569,.F.);
#14850=ADVANCED_FACE('',(#4215),#3570,.T.);
#14851=ADVANCED_FACE('',(#4216),#595,.T.);
#14852=ADVANCED_FACE('',(#4217),#596,.T.);
#14853=ADVANCED_FACE('',(#4218),#597,.T.);
#14854=ADVANCED_FACE('',(#4219),#3571,.T.);
#14855=ADVANCED_FACE('',(#4220),#598,.F.);
#14856=ADVANCED_FACE('',(#4221),#599,.F.);
#14857=ADVANCED_FACE('',(#4222),#3572,.T.);
#14858=ADVANCED_FACE('',(#4223),#600,.T.);
#14859=ADVANCED_FACE('',(#4224),#601,.T.);
#14860=ADVANCED_FACE('',(#4225),#602,.T.);
#14861=ADVANCED_FACE('',(#4226),#603,.F.);
#14862=ADVANCED_FACE('',(#4227),#604,.T.);
#14863=ADVANCED_FACE('',(#4228),#605,.F.);
#14864=ADVANCED_FACE('',(#4229),#3573,.T.);
#14865=ADVANCED_FACE('',(#4230),#606,.F.);
#14866=ADVANCED_FACE('',(#4231),#3574,.T.);
#14867=ADVANCED_FACE('',(#4232),#607,.T.);
#14868=ADVANCED_FACE('',(#4233),#608,.T.);
#14869=ADVANCED_FACE('',(#4234),#609,.T.);
#14870=ADVANCED_FACE('',(#4235),#610,.F.);
#14871=ADVANCED_FACE('',(#4236),#611,.T.);
#14872=ADVANCED_FACE('',(#4237),#612,.T.);
#14873=ADVANCED_FACE('',(#4238),#613,.T.);
#14874=ADVANCED_FACE('',(#4239),#614,.F.);
#14875=ADVANCED_FACE('',(#4240),#3575,.T.);
#14876=ADVANCED_FACE('',(#4241),#615,.T.);
#14877=ADVANCED_FACE('',(#4242),#616,.F.);
#14878=ADVANCED_FACE('',(#4243),#3576,.T.);
#14879=ADVANCED_FACE('',(#4244),#617,.F.);
#14880=ADVANCED_FACE('',(#4245),#618,.T.);
#14881=ADVANCED_FACE('',(#4246),#3577,.F.);
#14882=ADVANCED_FACE('',(#4247),#3578,.T.);
#14883=ADVANCED_FACE('',(#4248),#3579,.F.);
#14884=ADVANCED_FACE('',(#4249),#3580,.T.);
#14885=ADVANCED_FACE('',(#4250),#619,.T.);
#14886=ADVANCED_FACE('',(#4251),#620,.T.);
#14887=ADVANCED_FACE('',(#4252),#3581,.T.);
#14888=ADVANCED_FACE('',(#4253),#621,.F.);
#14889=ADVANCED_FACE('',(#4254),#622,.F.);
#14890=ADVANCED_FACE('',(#4255,#235),#623,.F.);
#14891=ADVANCED_FACE('',(#4256,#236),#624,.T.);
#14892=ADVANCED_FACE('',(#4257),#625,.F.);
#14893=ADVANCED_FACE('',(#4258),#626,.F.);
#14894=ADVANCED_FACE('',(#4259),#627,.F.);
#14895=ADVANCED_FACE('',(#4260),#628,.F.);
#14896=ADVANCED_FACE('',(#4261),#3582,.T.);
#14897=ADVANCED_FACE('',(#4262),#629,.F.);
#14898=ADVANCED_FACE('',(#4263),#3583,.T.);
#14899=ADVANCED_FACE('',(#4264),#630,.F.);
#14900=ADVANCED_FACE('',(#4265,#237),#631,.T.);
#14901=ADVANCED_FACE('',(#4266),#3584,.T.);
#14902=ADVANCED_FACE('',(#4267,#238),#632,.F.);
#14903=ADVANCED_FACE('',(#4268),#633,.F.);
#14904=ADVANCED_FACE('',(#4269),#634,.F.);
#14905=ADVANCED_FACE('',(#4270,#239),#635,.T.);
#14906=ADVANCED_FACE('',(#4271),#636,.F.);
#14907=ADVANCED_FACE('',(#4272),#3585,.T.);
#15198=CLOSED_SHELL('',(#14821,#14822,#14823,#14824,#14825,#14826,#14827,
#14828,#14829,#14830,#14831,#14832,#14833,#14834,#14835,#14836,#14837,#14838,
#14839,#14840,#14841,#14842,#14843,#14844,#14845,#14846,#14847,#14848,#14849,
#14850,#14851,#14852,#14853,#14854,#14855,#14856,#14857,#14858,#14859,#14860,
#14861,#14862,#14863,#14864,#14865,#14866,#14867,#14868,#14869,#14870,#14871,
#14872,#14873,#14874,#14875,#14876,#14877,#14878,#14879,#14880,#14881,#14882,
#14883,#14884,#14885,#14886,#14887,#14888,#14889,#14890,#14891,#14892,#14893,
#14894,#14895,#14896,#14897,#14898,#14899,#14900,#14901,#14902,#14903,#14904,
#14905,#14906,#14907));
#16214=AXIS2_PLACEMENT_3D('',#44531,#19456,#19457);
#16215=AXIS2_PLACEMENT_3D('',#44532,#19458,#19459);
#16216=AXIS2_PLACEMENT_3D('',#44537,#19461,#19462);
#16217=AXIS2_PLACEMENT_3D('',#44563,#19464,#19465);
#16218=AXIS2_PLACEMENT_3D('',#44566,#19467,#19468);
#16219=AXIS2_PLACEMENT_3D('',#44568,#19469,#19470);
#16220=AXIS2_PLACEMENT_3D('',#44571,#19472,#19473);
#16221=AXIS2_PLACEMENT_3D('',#44572,#19474,#19475);
#16222=AXIS2_PLACEMENT_3D('',#44577,#19477,#19478);
#16223=AXIS2_PLACEMENT_3D('',#44580,#19480,#19481);
#16224=AXIS2_PLACEMENT_3D('',#44582,#19482,#19483);
#16225=AXIS2_PLACEMENT_3D('',#44585,#19485,#19486);
#16226=AXIS2_PLACEMENT_3D('',#44586,#19487,#19488);
#16227=AXIS2_PLACEMENT_3D('',#44591,#19490,#19491);
#16228=AXIS2_PLACEMENT_3D('',#44617,#19493,#19494);
#16229=AXIS2_PLACEMENT_3D('',#44621,#19496,#19497);
#16230=AXIS2_PLACEMENT_3D('',#44646,#19499,#19500);
#16231=AXIS2_PLACEMENT_3D('',#44648,#19501,#19502);
#16232=AXIS2_PLACEMENT_3D('',#44651,#19504,#19505);
#16233=AXIS2_PLACEMENT_3D('',#44653,#19506,#19507);
#16234=AXIS2_PLACEMENT_3D('',#44656,#19509,#19510);
#16235=AXIS2_PLACEMENT_3D('',#44657,#19511,#19512);
#16236=AXIS2_PLACEMENT_3D('',#44659,#19513,#19514);
#16237=AXIS2_PLACEMENT_3D('',#44663,#19516,#19517);
#16238=AXIS2_PLACEMENT_3D('',#44689,#19519,#19520);
#16239=AXIS2_PLACEMENT_3D('',#44693,#19522,#19523);
#16240=AXIS2_PLACEMENT_3D('',#44696,#19525,#19526);
#16241=AXIS2_PLACEMENT_3D('',#44697,#19527,#19528);
#16242=AXIS2_PLACEMENT_3D('',#44702,#19530,#19531);
#16243=AXIS2_PLACEMENT_3D('',#44728,#19533,#19534);
#16244=AXIS2_PLACEMENT_3D('',#44732,#19536,#19537);
#16245=AXIS2_PLACEMENT_3D('',#44757,#19539,#19540);
#16246=AXIS2_PLACEMENT_3D('',#44758,#19541,#19542);
#16247=AXIS2_PLACEMENT_3D('',#44763,#19544,#19545);
#16248=AXIS2_PLACEMENT_3D('',#44789,#19547,#19548);
#16249=AXIS2_PLACEMENT_3D('',#44793,#19550,#19551);
#16250=AXIS2_PLACEMENT_3D('',#44818,#19553,#19554);
#16251=AXIS2_PLACEMENT_3D('',#44819,#19555,#19556);
#16252=AXIS2_PLACEMENT_3D('',#44821,#19557,#19558);
#16253=AXIS2_PLACEMENT_3D('',#44824,#19560,#19561);
#16254=AXIS2_PLACEMENT_3D('',#44825,#19562,#19563);
#16255=AXIS2_PLACEMENT_3D('',#44827,#19564,#19565);
#16256=AXIS2_PLACEMENT_3D('',#44830,#19567,#19568);
#16257=AXIS2_PLACEMENT_3D('',#44831,#19569,#19570);
#16258=AXIS2_PLACEMENT_3D('',#44833,#19571,#19572);
#16259=AXIS2_PLACEMENT_3D('',#44836,#19574,#19575);
#16260=AXIS2_PLACEMENT_3D('',#44837,#19576,#19577);
#16261=AXIS2_PLACEMENT_3D('',#44840,#19578,#19579);
#16262=AXIS2_PLACEMENT_3D('',#44844,#19581,#19582);
#16263=AXIS2_PLACEMENT_3D('',#44846,#19584,#19585);
#16264=AXIS2_PLACEMENT_3D('',#44848,#19586,#19587);
#16265=AXIS2_PLACEMENT_3D('',#44851,#19589,#19590);
#16266=AXIS2_PLACEMENT_3D('',#44852,#19591,#19592);
#16267=AXIS2_PLACEMENT_3D('',#44854,#19593,#19594);
#16268=AXIS2_PLACEMENT_3D('',#44857,#19596,#19597);
#16269=AXIS2_PLACEMENT_3D('',#44858,#19598,#19599);
#16270=AXIS2_PLACEMENT_3D('',#44860,#19600,#19601);
#16271=AXIS2_PLACEMENT_3D('',#44864,#19603,#19604);
#16272=AXIS2_PLACEMENT_3D('',#44868,#19606,#19607);
#16273=AXIS2_PLACEMENT_3D('',#44871,#19609,#19610);
#16274=AXIS2_PLACEMENT_3D('',#44872,#19611,#19612);
#16275=AXIS2_PLACEMENT_3D('',#44874,#19613,#19614);
#16276=AXIS2_PLACEMENT_3D('',#44877,#19616,#19617);
#16277=AXIS2_PLACEMENT_3D('',#44878,#19618,#19619);
#16278=AXIS2_PLACEMENT_3D('',#44880,#19620,#19621);
#16279=AXIS2_PLACEMENT_3D('',#44883,#19623,#19624);
#16280=AXIS2_PLACEMENT_3D('',#44884,#19625,#19626);
#16281=AXIS2_PLACEMENT_3D('',#44886,#19627,#19628);
#16282=AXIS2_PLACEMENT_3D('',#44890,#19630,#19631);
#16283=AXIS2_PLACEMENT_3D('',#44894,#19633,#19634);
#16284=AXIS2_PLACEMENT_3D('',#44897,#19636,#19637);
#16285=AXIS2_PLACEMENT_3D('',#44898,#19638,#19639);
#16286=AXIS2_PLACEMENT_3D('',#44900,#19640,#19641);
#16287=AXIS2_PLACEMENT_3D('',#44902,#19642,#19643);
#16288=AXIS2_PLACEMENT_3D('',#44904,#19645,#19646);
#16289=AXIS2_PLACEMENT_3D('',#44906,#19647,#19648);
#16290=AXIS2_PLACEMENT_3D('',#44909,#19650,#19651);
#16291=AXIS2_PLACEMENT_3D('',#44910,#19652,#19653);
#16292=AXIS2_PLACEMENT_3D('',#44911,#19654,#19655);
#16293=AXIS2_PLACEMENT_3D('',#44912,#19656,#19657);
#16294=AXIS2_PLACEMENT_3D('',#44914,#19658,#19659);
#16295=AXIS2_PLACEMENT_3D('',#44917,#19661,#19662);
#16296=AXIS2_PLACEMENT_3D('',#44918,#19663,#19664);
#16297=AXIS2_PLACEMENT_3D('',#44919,#19665,#19666);
#16298=AXIS2_PLACEMENT_3D('',#44922,#19669,#19670);
#16299=AXIS2_PLACEMENT_3D('',#44925,#19673,#19674);
#16300=AXIS2_PLACEMENT_3D('',#44928,#19675,#19676);
#16301=AXIS2_PLACEMENT_3D('',#44932,#19678,#19679);
#16302=AXIS2_PLACEMENT_3D('',#44934,#19681,#19682);
#16303=AXIS2_PLACEMENT_3D('',#44938,#19686,#19687);
#16304=AXIS2_PLACEMENT_3D('',#44942,#19689,#19690);
#16305=AXIS2_PLACEMENT_3D('',#44944,#19692,#19693);
#16306=AXIS2_PLACEMENT_3D('',#44945,#19694,#19695);
#16307=AXIS2_PLACEMENT_3D('',#44952,#19700,#19701);
#16308=AXIS2_PLACEMENT_3D('',#44956,#19703,#19704);
#16309=AXIS2_PLACEMENT_3D('',#44958,#19706,#19707);
#16310=AXIS2_PLACEMENT_3D('',#44960,#19709,#19710);
#16311=AXIS2_PLACEMENT_3D('',#44962,#19712,#19713);
#16312=AXIS2_PLACEMENT_3D('',#44968,#19717,#19718);
#16313=AXIS2_PLACEMENT_3D('',#44971,#19721,#19722);
#16314=AXIS2_PLACEMENT_3D('',#44972,#19723,#19724);
#16315=AXIS2_PLACEMENT_3D('',#44973,#19725,#19726);
#16316=AXIS2_PLACEMENT_3D('',#44974,#19727,#19728);
#16317=AXIS2_PLACEMENT_3D('',#44977,#19731,#19732);
#16318=AXIS2_PLACEMENT_3D('',#44979,#19733,#19734);
#16319=AXIS2_PLACEMENT_3D('',#44982,#19736,#19737);
#16320=AXIS2_PLACEMENT_3D('',#44983,#19738,#19739);
#16321=AXIS2_PLACEMENT_3D('',#44989,#19743,#19744);
#16322=AXIS2_PLACEMENT_3D('',#44990,#19745,#19746);
#16323=AXIS2_PLACEMENT_3D('',#44996,#19750,#19751);
#16324=AXIS2_PLACEMENT_3D('',#45002,#19755,#19756);
#16325=AXIS2_PLACEMENT_3D('',#45004,#19758,#19759);
#16326=AXIS2_PLACEMENT_3D('',#45005,#19760,#19761);
#16327=AXIS2_PLACEMENT_3D('',#45007,#19763,#19764);
#16328=AXIS2_PLACEMENT_3D('',#45008,#19765,#19766);
#16329=AXIS2_PLACEMENT_3D('',#45009,#19767,#19768);
#16330=AXIS2_PLACEMENT_3D('',#45012,#19771,#19772);
#16331=AXIS2_PLACEMENT_3D('',#45015,#19773,#19774);
#16332=AXIS2_PLACEMENT_3D('',#45019,#19776,#19777);
#16333=AXIS2_PLACEMENT_3D('',#45021,#19779,#19780);
#16334=AXIS2_PLACEMENT_3D('',#45027,#19784,#19785);
#16335=AXIS2_PLACEMENT_3D('',#45029,#19786,#19787);
#16336=AXIS2_PLACEMENT_3D('',#45037,#19793,#19794);
#16337=AXIS2_PLACEMENT_3D('',#45043,#19798,#19799);
#16338=AXIS2_PLACEMENT_3D('',#45045,#19801,#19802);
#16339=AXIS2_PLACEMENT_3D('',#45048,#19804,#19805);
#16340=AXIS2_PLACEMENT_3D('',#45051,#19808,#19809);
#16341=AXIS2_PLACEMENT_3D('',#45054,#19812,#19813);
#16342=AXIS2_PLACEMENT_3D('',#45056,#19815,#19816);
#16343=AXIS2_PLACEMENT_3D('',#45057,#19817,#19818);
#16344=AXIS2_PLACEMENT_3D('',#45058,#19819,#19820);
#16345=AXIS2_PLACEMENT_3D('',#45061,#19823,#19824);
#16346=AXIS2_PLACEMENT_3D('',#45064,#19827,#19828);
#16347=AXIS2_PLACEMENT_3D('',#45067,#19829,#19830);
#16348=AXIS2_PLACEMENT_3D('',#45071,#19832,#19833);
#16349=AXIS2_PLACEMENT_3D('',#45073,#19835,#19836);
#16350=AXIS2_PLACEMENT_3D('',#45077,#19840,#19841);
#16351=AXIS2_PLACEMENT_3D('',#45081,#19843,#19844);
#16352=AXIS2_PLACEMENT_3D('',#45083,#19846,#19847);
#16353=AXIS2_PLACEMENT_3D('',#45084,#19848,#19849);
#16354=AXIS2_PLACEMENT_3D('',#45088,#19851,#19852);
#16355=AXIS2_PLACEMENT_3D('',#45090,#19854,#19855);
#16356=AXIS2_PLACEMENT_3D('',#45092,#19857,#19858);
#16357=AXIS2_PLACEMENT_3D('',#45093,#19859,#19860);
#16358=AXIS2_PLACEMENT_3D('',#45096,#19863,#19864);
#16359=AXIS2_PLACEMENT_3D('',#45097,#19865,#19866);
#16360=AXIS2_PLACEMENT_3D('',#45098,#19867,#19868);
#16361=AXIS2_PLACEMENT_3D('',#45099,#19869,#19870);
#16362=AXIS2_PLACEMENT_3D('',#45100,#19871,#19872);
#16363=AXIS2_PLACEMENT_3D('',#45101,#19873,#19874);
#16364=AXIS2_PLACEMENT_3D('',#45102,#19875,#19876);
#16365=AXIS2_PLACEMENT_3D('',#45103,#19877,#19878);
#16366=AXIS2_PLACEMENT_3D('',#45112,#19883,#19884);
#16367=AXIS2_PLACEMENT_3D('',#45118,#19888,#19889);
#16368=AXIS2_PLACEMENT_3D('',#45127,#19894,#19895);
#16369=AXIS2_PLACEMENT_3D('',#45129,#19896,#19897);
#16370=AXIS2_PLACEMENT_3D('',#45132,#19899,#19900);
#16371=AXIS2_PLACEMENT_3D('',#45133,#19901,#19902);
#16372=AXIS2_PLACEMENT_3D('',#45139,#19906,#19907);
#16373=AXIS2_PLACEMENT_3D('',#45141,#19908,#19909);
#16374=AXIS2_PLACEMENT_3D('',#45144,#19911,#19912);
#16375=AXIS2_PLACEMENT_3D('',#45145,#19913,#19914);
#16376=AXIS2_PLACEMENT_3D('',#45151,#19918,#19919);
#16377=AXIS2_PLACEMENT_3D('',#45153,#19920,#19921);
#16378=AXIS2_PLACEMENT_3D('',#45156,#19923,#19924);
#16379=AXIS2_PLACEMENT_3D('',#45157,#19925,#19926);
#16380=AXIS2_PLACEMENT_3D('',#45160,#19928,#19929);
#16381=AXIS2_PLACEMENT_3D('',#45161,#19930,#19931);
#16382=AXIS2_PLACEMENT_3D('',#45164,#19933,#19934);
#16383=AXIS2_PLACEMENT_3D('',#45168,#19937,#19938);
#16384=AXIS2_PLACEMENT_3D('',#45170,#19940,#19941);
#16385=AXIS2_PLACEMENT_3D('',#45174,#19944,#19945);
#16386=AXIS2_PLACEMENT_3D('',#45176,#19947,#19948);
#16387=AXIS2_PLACEMENT_3D('',#45177,#19949,#19950);
#19456=DIRECTION('axis',(0.,0.,1.));
#19457=DIRECTION('refdir',(1.,0.,0.));
#19458=DIRECTION('center_axis',(-0.109509747813017,0.,0.993985721795806));
#19459=DIRECTION('ref_axis',(-0.993985721795806,0.,-0.109509747813017));
#19460=DIRECTION('',(0.109509747813017,0.,-0.993985721795806));
#19461=DIRECTION('center_axis',(0.109509747813016,0.,-0.993985721795806));
#19462=DIRECTION('ref_axis',(-0.993985721795806,0.,-0.109509747813016));
#19463=DIRECTION('',(-0.109509747813016,0.,0.993985721795806));
#19464=DIRECTION('center_axis',(-0.109509747813016,0.,0.993985721795806));
#19465=DIRECTION('ref_axis',(-0.993985721795806,0.,-0.109509747813016));
#19466=DIRECTION('',(0.109509747813017,0.,-0.993985721795806));
#19467=DIRECTION('center_axis',(0.109509747813017,0.,-0.993985721795806));
#19468=DIRECTION('ref_axis',(0.993985721795806,0.,0.109509747813017));
#19469=DIRECTION('center_axis',(-0.109509747813016,0.,0.993985721795806));
#19470=DIRECTION('ref_axis',(-0.993985721795806,0.,-0.109509747813016));
#19471=DIRECTION('',(-0.109509747813016,-5.79756587691265E-17,0.993985721795806));
#19472=DIRECTION('center_axis',(0.109509747813016,0.,-0.993985721795806));
#19473=DIRECTION('ref_axis',(-6.66524446162044E-16,1.,-7.34325679030328E-17));
#19474=DIRECTION('center_axis',(-0.109509747813017,0.,0.993985721795806));
#19475=DIRECTION('ref_axis',(-0.993985721795806,0.,-0.109509747813017));
#19476=DIRECTION('',(0.109509747813017,0.,-0.993985721795806));
#19477=DIRECTION('center_axis',(0.109509747813016,0.,-0.993985721795806));
#19478=DIRECTION('ref_axis',(-0.993985721795806,0.,-0.109509747813016));
#19479=DIRECTION('',(-0.109509747813016,5.79756587691264E-17,0.993985721795806));
#19480=DIRECTION('center_axis',(0.109509747813016,0.,-0.993985721795806));
#19481=DIRECTION('ref_axis',(-0.993985721795806,0.,-0.109509747813016));
#19482=DIRECTION('center_axis',(0.109509747813016,0.,-0.993985721795806));
#19483=DIRECTION('ref_axis',(-6.66524446162044E-16,1.,-7.34325679030328E-17));
#19484=DIRECTION('',(0.109509747813016,3.61400724161835E-16,-0.993985721795806));
#19485=DIRECTION('center_axis',(0.109509747813016,0.,-0.993985721795806));
#19486=DIRECTION('ref_axis',(-6.66524446162044E-16,1.,-7.34325679030328E-17));
#19487=DIRECTION('center_axis',(-0.109509747813017,0.,0.993985721795806));
#19488=DIRECTION('ref_axis',(-0.993985721795806,0.,-0.109509747813017));
#19489=DIRECTION('',(0.109509747813017,0.,-0.993985721795806));
#19490=DIRECTION('center_axis',(0.109509747813016,0.,-0.993985721795806));
#19491=DIRECTION('ref_axis',(-0.993985721795806,0.,-0.109509747813016));
#19492=DIRECTION('',(-0.109509747813016,0.,0.993985721795806));
#19493=DIRECTION('center_axis',(-0.109509747813016,0.,0.993985721795806));
#19494=DIRECTION('ref_axis',(0.936831271488445,-0.334206918693375,0.103212907423556));
#19495=DIRECTION('',(0.109509747813017,0.,-0.993985721795806));
#19496=DIRECTION('center_axis',(-0.109509747813016,0.,0.993985721795806));
#19497=DIRECTION('ref_axis',(-0.993985721795806,0.,-0.109509747813016));
#19498=DIRECTION('',(0.109509747813016,0.,-0.993985721795806));
#19499=DIRECTION('center_axis',(0.109509747813016,0.,-0.993985721795806));
#19500=DIRECTION('ref_axis',(-0.993985721795806,0.,-0.109509747813016));
#19501=DIRECTION('center_axis',(0.109509747813016,0.,-0.993985721795806));
#19502=DIRECTION('ref_axis',(-6.66524446162044E-16,1.,-7.34325679030328E-17));
#19503=DIRECTION('',(-0.109509747813016,-5.79756587691265E-17,0.993985721795806));
#19504=DIRECTION('center_axis',(-0.109509747813016,0.,0.993985721795806));
#19505=DIRECTION('ref_axis',(-0.993985721795806,0.,-0.109509747813016));
#19506=DIRECTION('center_axis',(-0.109509747813016,0.,0.993985721795806));
#19507=DIRECTION('ref_axis',(0.936831271488445,-0.334206918693375,0.103212907423556));
#19508=DIRECTION('',(-0.109509747813016,-5.79756587691265E-17,0.993985721795806));
#19509=DIRECTION('center_axis',(0.109509747813016,0.,-0.993985721795806));
#19510=DIRECTION('ref_axis',(-7.61742224185193E-16,1.,-8.39229347463232E-17));
#19511=DIRECTION('center_axis',(-0.109509747813017,0.,0.993985721795806));
#19512=DIRECTION('ref_axis',(-0.993985721795806,0.,-0.109509747813017));
#19513=DIRECTION('center_axis',(-0.109509747813016,0.,0.993985721795806));
#19514=DIRECTION('ref_axis',(-0.993985721795806,0.,-0.109509747813016));
#19515=DIRECTION('',(0.109509747813017,0.,-0.993985721795806));
#19516=DIRECTION('center_axis',(-0.109509747813016,0.,0.993985721795806));
#19517=DIRECTION('ref_axis',(0.936831271488445,-0.334206918693375,0.103212907423556));
#19518=DIRECTION('',(0.109509747813016,0.,-0.993985721795806));
#19519=DIRECTION('center_axis',(0.109509747813016,0.,-0.993985721795806));
#19520=DIRECTION('ref_axis',(-0.993985721795806,0.,-0.109509747813016));
#19521=DIRECTION('',(0.109509747813017,0.,-0.993985721795806));
#19522=DIRECTION('center_axis',(0.109509747813016,0.,-0.993985721795806));
#19523=DIRECTION('ref_axis',(-7.61742224185193E-16,1.,-8.39229347463232E-17));
#19524=DIRECTION('',(-0.109509747813016,-5.79756587691265E-17,0.993985721795806));
#19525=DIRECTION('center_axis',(-0.109509747813016,0.,0.993985721795806));
#19526=DIRECTION('ref_axis',(0.936831271488445,-0.334206918693375,0.103212907423556));
#19527=DIRECTION('center_axis',(0.109509747813016,0.,-0.993985721795806));
#19528=DIRECTION('ref_axis',(0.993985721795806,0.,0.109509747813016));
#19529=DIRECTION('',(-0.109509747813016,0.,0.993985721795806));
#19530=DIRECTION('center_axis',(-0.109509747813016,0.,0.993985721795806));
#19531=DIRECTION('ref_axis',(-0.993985721795806,0.,-0.109509747813016));
#19532=DIRECTION('',(0.109509747813015,7.50701870275913E-16,-0.993985721795806));
#19533=DIRECTION('center_axis',(0.109509747813016,0.,-0.993985721795806));
#19534=DIRECTION('ref_axis',(0.936831271488447,0.33420691869337,0.103212907423556));
#19535=DIRECTION('',(0.109509747813016,3.00462919747432E-16,-0.993985721795806));
#19536=DIRECTION('center_axis',(0.109509747813016,0.,-0.993985721795806));
#19537=DIRECTION('ref_axis',(0.936831271488447,0.33420691869337,0.103212907423556));
#19538=DIRECTION('',(-0.109509747813016,0.,0.993985721795806));
#19539=DIRECTION('center_axis',(-0.109509747813016,0.,0.993985721795806));
#19540=DIRECTION('ref_axis',(-0.993985721795806,0.,-0.109509747813016));
#19541=DIRECTION('center_axis',(0.109509747813016,0.,-0.993985721795806));
#19542=DIRECTION('ref_axis',(0.993985721795806,0.,0.109509747813016));
#19543=DIRECTION('',(-0.109509747813016,0.,0.993985721795806));
#19544=DIRECTION('center_axis',(-0.109509747813016,0.,0.993985721795806));
#19545=DIRECTION('ref_axis',(0.936831271488445,-0.334206918693375,0.103212907423556));
#19546=DIRECTION('',(0.109509747813015,7.50701870275913E-16,-0.993985721795806));
#19547=DIRECTION('center_axis',(0.109509747813016,0.,-0.993985721795806));
#19548=DIRECTION('ref_axis',(0.936831271488447,0.33420691869337,0.103212907423556));
#19549=DIRECTION('',(0.109509747813016,3.00462919747432E-16,-0.993985721795806));
#19550=DIRECTION('center_axis',(0.109509747813016,0.,-0.993985721795806));
#19551=DIRECTION('ref_axis',(0.936831271488447,0.33420691869337,0.103212907423556));
#19552=DIRECTION('',(-0.109509747813016,0.,0.993985721795806));
#19553=DIRECTION('center_axis',(-0.109509747813016,0.,0.993985721795806));
#19554=DIRECTION('ref_axis',(0.936831271488445,-0.334206918693375,0.103212907423556));
#19555=DIRECTION('center_axis',(0.109509747813016,0.,-0.993985721795806));
#19556=DIRECTION('ref_axis',(0.993985721795806,0.,0.109509747813016));
#19557=DIRECTION('center_axis',(0.109509747813016,0.,-0.993985721795806));
#19558=DIRECTION('ref_axis',(0.993985721795806,0.,0.109509747813016));
#19559=DIRECTION('',(0.109509747813016,0.,-0.993985721795806));
#19560=DIRECTION('center_axis',(0.109509747813016,0.,-0.993985721795806));
#19561=DIRECTION('ref_axis',(0.993985721795806,0.,0.109509747813016));
#19562=DIRECTION('center_axis',(0.109509747813016,0.,-0.993985721795806));
#19563=DIRECTION('ref_axis',(0.993985721795806,0.,0.109509747813016));
#19564=DIRECTION('center_axis',(-0.109509747813016,0.,0.993985721795806));
#19565=DIRECTION('ref_axis',(0.993985721795806,0.,0.109509747813016));
#19566=DIRECTION('',(-0.109509747813016,0.,0.993985721795806));
#19567=DIRECTION('center_axis',(0.109509747813016,0.,-0.993985721795806));
#19568=DIRECTION('ref_axis',(-0.993985721795806,0.,-0.109509747813016));
#19569=DIRECTION('center_axis',(-0.109509747813016,0.,0.993985721795806));
#19570=DIRECTION('ref_axis',(-0.993985721795806,0.,-0.109509747813016));
#19571=DIRECTION('center_axis',(-0.109509747813016,0.,0.993985721795806));
#19572=DIRECTION('ref_axis',(0.993985721795806,0.,0.109509747813016));
#19573=DIRECTION('',(-0.109509747813016,0.,0.993985721795806));
#19574=DIRECTION('center_axis',(-0.109509747813016,0.,0.993985721795806));
#19575=DIRECTION('ref_axis',(0.993985721795806,0.,0.109509747813016));
#19576=DIRECTION('center_axis',(-0.109509747813016,0.,0.993985721795806));
#19577=DIRECTION('ref_axis',(-0.993985721795806,0.,-0.109509747813016));
#19578=DIRECTION('center_axis',(-0.109509747813016,0.,0.993985721795806));
#19579=DIRECTION('ref_axis',(-0.993985721795806,0.,-0.109509747813016));
#19580=DIRECTION('',(-0.109509747813016,5.79756587691264E-17,0.993985721795806));
#19581=DIRECTION('center_axis',(-0.109509747813016,0.,0.993985721795806));
#19582=DIRECTION('ref_axis',(-0.993985721795806,0.,-0.109509747813016));
#19583=DIRECTION('',(-0.109509747813016,-1.50231459873716E-16,0.993985721795806));
#19584=DIRECTION('center_axis',(-0.109509747813016,0.,0.993985721795806));
#19585=DIRECTION('ref_axis',(-0.993985721795806,0.,-0.109509747813016));
#19586=DIRECTION('center_axis',(-0.109509747813016,0.,0.993985721795806));
#19587=DIRECTION('ref_axis',(-0.936831271488455,0.334206918693347,-0.103212907423557));
#19588=DIRECTION('',(-0.109509747813016,1.50231459873716E-16,0.993985721795806));
#19589=DIRECTION('center_axis',(0.109509747813016,0.,-0.993985721795806));
#19590=DIRECTION('ref_axis',(-0.496992860897901,-0.86602540378444,-0.0547548739065078));
#19591=DIRECTION('center_axis',(-0.109509747813016,0.,0.993985721795806));
#19592=DIRECTION('ref_axis',(-0.993985721795806,0.,-0.109509747813016));
#19593=DIRECTION('center_axis',(0.109509747813016,0.,-0.993985721795806));
#19594=DIRECTION('ref_axis',(-0.496992860897901,-0.86602540378444,-0.0547548739065078));
#19595=DIRECTION('',(-0.109509747813016,1.50231459873716E-16,0.993985721795806));
#19596=DIRECTION('center_axis',(-0.109509747813016,0.,0.993985721795806));
#19597=DIRECTION('ref_axis',(-0.936831271488455,0.334206918693348,-0.103212907423557));
#19598=DIRECTION('center_axis',(0.109509747813016,0.,-0.993985721795806));
#19599=DIRECTION('ref_axis',(0.993985721795806,0.,0.109509747813016));
#19600=DIRECTION('center_axis',(-0.109509747813016,0.,0.993985721795806));
#19601=DIRECTION('ref_axis',(0.936831271488445,-0.334206918693375,0.103212907423556));
#19602=DIRECTION('',(0.109509747813016,1.15951317538253E-16,-0.993985721795806));
#19603=DIRECTION('center_axis',(0.109509747813016,0.,-0.993985721795806));
#19604=DIRECTION('ref_axis',(-6.23243637969703E-16,1.,-6.86642193379008E-17));
#19605=DIRECTION('',(-0.109509747813016,0.,0.993985721795806));
#19606=DIRECTION('center_axis',(0.109509747813016,0.,-0.993985721795806));
#19607=DIRECTION('ref_axis',(-6.23243637969703E-16,1.,-6.86642193379008E-17));
#19608=DIRECTION('',(0.109509747813016,1.15951317538253E-16,-0.993985721795806));
#19609=DIRECTION('center_axis',(-0.109509747813016,0.,0.993985721795806));
#19610=DIRECTION('ref_axis',(0.936831271488445,-0.334206918693375,0.103212907423556));
#19611=DIRECTION('center_axis',(-0.109509747813016,0.,0.993985721795806));
#19612=DIRECTION('ref_axis',(-0.993985721795806,0.,-0.109509747813016));
#19613=DIRECTION('center_axis',(-0.109509747813016,0.,0.993985721795806));
#19614=DIRECTION('ref_axis',(-0.936831271488455,0.334206918693348,-0.103212907423557));
#19615=DIRECTION('',(-0.109509747813016,1.50231459873716E-16,0.993985721795806));
#19616=DIRECTION('center_axis',(0.109509747813016,0.,-0.993985721795806));
#19617=DIRECTION('ref_axis',(-0.496992860897901,-0.86602540378444,-0.0547548739065078));
#19618=DIRECTION('center_axis',(-0.109509747813016,0.,0.993985721795806));
#19619=DIRECTION('ref_axis',(-0.993985721795806,0.,-0.109509747813016));
#19620=DIRECTION('center_axis',(0.109509747813016,0.,-0.993985721795806));
#19621=DIRECTION('ref_axis',(-0.496992860897901,-0.86602540378444,-0.0547548739065078));
#19622=DIRECTION('',(-0.109509747813016,1.50231459873716E-16,0.993985721795806));
#19623=DIRECTION('center_axis',(-0.109509747813016,0.,0.993985721795806));
#19624=DIRECTION('ref_axis',(-0.936831271488455,0.334206918693348,-0.103212907423557));
#19625=DIRECTION('center_axis',(0.109509747813016,0.,-0.993985721795806));
#19626=DIRECTION('ref_axis',(0.993985721795806,0.,0.109509747813016));
#19627=DIRECTION('center_axis',(-0.109509747813016,0.,0.993985721795806));
#19628=DIRECTION('ref_axis',(-0.993985721795806,0.,-0.109509747813016));
#19629=DIRECTION('',(0.109509747813016,1.15951317538253E-16,-0.993985721795806));
#19630=DIRECTION('center_axis',(0.109509747813016,0.,-0.993985721795806));
#19631=DIRECTION('ref_axis',(-5.4533818322349E-16,1.,-6.00811919206632E-17));
#19632=DIRECTION('',(-0.109509747813016,0.,0.993985721795806));
#19633=DIRECTION('center_axis',(0.109509747813016,0.,-0.993985721795806));
#19634=DIRECTION('ref_axis',(-5.4533818322349E-16,1.,-6.00811919206632E-17));
#19635=DIRECTION('',(0.109509747813016,1.15951317538253E-16,-0.993985721795806));
#19636=DIRECTION('center_axis',(-0.109509747813016,0.,0.993985721795806));
#19637=DIRECTION('ref_axis',(-0.993985721795806,0.,-0.109509747813016));
#19638=DIRECTION('center_axis',(-0.109509747813016,0.,0.993985721795806));
#19639=DIRECTION('ref_axis',(-0.993985721795806,0.,-0.109509747813016));
#19640=DIRECTION('center_axis',(-0.109509747813016,0.,0.993985721795806));
#19641=DIRECTION('ref_axis',(-0.993985721795806,0.,-0.109509747813016));
#19642=DIRECTION('center_axis',(-0.109509747813016,0.,0.993985721795806));
#19643=DIRECTION('ref_axis',(-0.993985721795806,0.,-0.109509747813016));
#19644=DIRECTION('',(-0.109509747813016,-1.50231459873716E-16,0.993985721795806));
#19645=DIRECTION('center_axis',(-0.109509747813017,0.,0.993985721795806));
#19646=DIRECTION('ref_axis',(-0.993985721795806,0.,-0.109509747813017));
#19647=DIRECTION('center_axis',(0.109509747813017,0.,-0.993985721795806));
#19648=DIRECTION('ref_axis',(-0.993985721795806,0.,-0.109509747813017));
#19649=DIRECTION('',(-0.109509747813017,0.,0.993985721795806));
#19650=DIRECTION('center_axis',(0.109509747813017,0.,-0.993985721795806));
#19651=DIRECTION('ref_axis',(-0.993985721795806,0.,-0.109509747813017));
#19652=DIRECTION('center_axis',(-0.109509747813017,0.,0.993985721795806));
#19653=DIRECTION('ref_axis',(-0.993985721795806,0.,-0.109509747813017));
#19654=DIRECTION('center_axis',(0.109509747813016,0.,-0.993985721795806));
#19655=DIRECTION('ref_axis',(-0.993985721795806,0.,-0.109509747813016));
#19656=DIRECTION('center_axis',(0.109509747813016,0.,-0.993985721795806));
#19657=DIRECTION('ref_axis',(-0.993985721795806,0.,-0.109509747813016));
#19658=DIRECTION('center_axis',(0.109509747813016,0.,-0.993985721795806));
#19659=DIRECTION('ref_axis',(-7.61742224185193E-16,1.,-8.39229347463232E-17));
#19660=DIRECTION('',(0.109509747813016,3.61400724161835E-16,-0.993985721795806));
#19661=DIRECTION('center_axis',(0.109509747813016,0.,-0.993985721795806));
#19662=DIRECTION('ref_axis',(-7.61742224185193E-16,1.,-8.39229347463232E-17));
#19663=DIRECTION('center_axis',(0.109509747813017,0.,-0.993985721795806));
#19664=DIRECTION('ref_axis',(0.,-1.,0.));
#19665=DIRECTION('center_axis',(0.645221227515378,0.760681545236145,0.0710855421355126));
#19666=DIRECTION('ref_axis',(0.109509747813016,-3.16883939248426E-18,-0.993985721795806));
#19667=DIRECTION('',(-0.756106594798299,0.64912524734226,-0.0833020441848256));
#19668=DIRECTION('',(0.756106594798299,-0.64912524734226,0.0833020441848256));
#19669=DIRECTION('center_axis',(-0.645221227515378,-0.760681545236145,-0.0710855421355126));
#19670=DIRECTION('ref_axis',(-0.756106594798299,0.64912524734226,-0.0833020441848256));
#19671=DIRECTION('',(-0.756106594798299,0.64912524734226,-0.0833020441848256));
#19672=DIRECTION('',(0.756106594798299,-0.64912524734226,0.0833020441848256));
#19673=DIRECTION('center_axis',(-0.496992860897903,0.866025403784439,-0.054754873906508));
#19674=DIRECTION('ref_axis',(0.86081688607418,0.5,0.0948382235681014));
#19675=DIRECTION('center_axis',(-0.496992860897903,0.866025403784439,-0.0547548739065078));
#19676=DIRECTION('ref_axis',(-0.86081688607418,-0.5,-0.0948382235681014));
#19677=DIRECTION('',(-0.496992860897903,0.866025403784439,-0.054754873906508));
#19678=DIRECTION('center_axis',(0.496992860897903,-0.866025403784439,0.0547548739065076));
#19679=DIRECTION('ref_axis',(0.86081688607418,0.5,0.0948382235681014));
#19680=DIRECTION('',(0.496992860897903,-0.866025403784439,0.054754873906508));
#19681=DIRECTION('center_axis',(0.109509747813016,0.,-0.993985721795806));
#19682=DIRECTION('ref_axis',(0.,-1.,0.));
#19683=DIRECTION('',(0.756106594798299,-0.64912524734226,0.0833020441848256));
#19684=DIRECTION('',(-0.86081688607418,-0.5,-0.0948382235680992));
#19685=DIRECTION('',(-0.86081688607418,-0.5,-0.0948382235680992));
#19686=DIRECTION('center_axis',(-0.496992860897903,0.866025403784439,-0.0547548739065078));
#19687=DIRECTION('ref_axis',(-0.109509747813016,-8.62567737696967E-18,0.993985721795806));
#19688=DIRECTION('',(-0.109509747813016,-1.50231459873716E-16,0.993985721795806));
#19689=DIRECTION('center_axis',(-0.496992860897903,0.866025403784439,-0.0547548739065078));
#19690=DIRECTION('ref_axis',(-0.86081688607418,-0.5,-0.0948382235681014));
#19691=DIRECTION('',(-0.86081688607418,-0.5,-0.0948382235680992));
#19692=DIRECTION('center_axis',(-0.756106594798299,0.64912524734226,-0.0833020441848257));
#19693=DIRECTION('ref_axis',(0.645221227515377,0.760681545236146,0.0710855421355155));
#19694=DIRECTION('center_axis',(0.109509747813016,0.,-0.993985721795806));
#19695=DIRECTION('ref_axis',(0.,-1.,0.));
#19696=DIRECTION('',(0.756106594798299,-0.64912524734226,0.0833020441848257));
#19697=DIRECTION('',(-0.86081688607418,0.5,-0.0948382235680992));
#19698=DIRECTION('',(-0.496992860897903,-0.866025403784439,-0.054754873906508));
#19699=DIRECTION('',(-0.86081688607418,0.5,-0.0948382235680992));
#19700=DIRECTION('center_axis',(0.496992860897903,-0.866025403784439,0.054754873906508));
#19701=DIRECTION('ref_axis',(-0.86081688607418,-0.5,-0.0948382235681014));
#19702=DIRECTION('',(-0.496992860897903,0.866025403784439,-0.054754873906508));
#19703=DIRECTION('center_axis',(0.496992860897903,-0.866025403784439,0.0547548739065076));
#19704=DIRECTION('ref_axis',(0.86081688607418,0.5,0.0948382235681014));
#19705=DIRECTION('',(0.496992860897903,-0.866025403784439,0.054754873906508));
#19706=DIRECTION('center_axis',(-0.756106594798299,0.64912524734226,-0.0833020441848257));
#19707=DIRECTION('ref_axis',(0.645221227515377,0.760681545236146,0.0710855421355154));
#19708=DIRECTION('',(-0.756106594798299,0.64912524734226,-0.0833020441848257));
#19709=DIRECTION('center_axis',(0.756106594798299,-0.64912524734226,0.0833020441848257));
#19710=DIRECTION('ref_axis',(-0.645221227515377,-0.760681545236146,-0.0710855421355154));
#19711=DIRECTION('',(-0.756106594798299,0.64912524734226,-0.0833020441848256));
#19712=DIRECTION('center_axis',(-0.109509747813016,0.,0.993985721795806));
#19713=DIRECTION('ref_axis',(0.993985721795806,0.,0.109509747813016));
#19714=DIRECTION('',(-0.86081688607418,0.5,-0.0948382235680992));
#19715=DIRECTION('',(0.496992860897903,0.866025403784439,0.054754873906508));
#19716=DIRECTION('',(-0.86081688607418,0.5,-0.0948382235680992));
#19717=DIRECTION('center_axis',(0.496992860897903,-0.866025403784439,0.0547548739065076));
#19718=DIRECTION('ref_axis',(0.109509747813016,4.04398041928102E-16,-0.993985721795806));
#19719=DIRECTION('',(-0.86081688607418,-0.5,-0.0948382235680992));
#19720=DIRECTION('',(0.109509747813016,3.00462919747432E-16,-0.993985721795806));
#19721=DIRECTION('center_axis',(0.109509747813016,0.,-0.993985721795806));
#19722=DIRECTION('ref_axis',(0.,-1.,0.));
#19723=DIRECTION('center_axis',(-0.756106594798299,0.64912524734226,-0.0833020441848257));
#19724=DIRECTION('ref_axis',(0.645221227515377,0.760681545236146,0.0710855421355155));
#19725=DIRECTION('center_axis',(-0.86081688607418,-0.5,-0.0948382235680992));
#19726=DIRECTION('ref_axis',(-0.496992860897903,0.866025403784439,-0.054754873906508));
#19727=DIRECTION('center_axis',(-0.993985721795806,6.12303176911189E-17,
-0.109509747813016));
#19728=DIRECTION('ref_axis',(-0.109509747813016,-4.27307853354592E-34,0.993985721795806));
#19729=DIRECTION('',(-3.7115920228551E-17,-1.,-2.22241612446982E-16));
#19730=DIRECTION('',(1.08354344120878E-16,1.,-4.24367274947369E-16));
#19731=DIRECTION('center_axis',(-0.496992860897903,-0.866025403784439,-0.054754873906508));
#19732=DIRECTION('ref_axis',(-0.86081688607418,0.5,-0.0948382235681014));
#19733=DIRECTION('center_axis',(-0.496992860897903,-0.866025403784439,-0.0547548739065078));
#19734=DIRECTION('ref_axis',(0.86081688607418,-0.5,0.0948382235681014));
#19735=DIRECTION('',(-0.496992860897903,-0.866025403784439,-0.054754873906508));
#19736=DIRECTION('center_axis',(0.496992860897903,0.866025403784439,0.0547548739065076));
#19737=DIRECTION('ref_axis',(-0.86081688607418,0.5,-0.0948382235681014));
#19738=DIRECTION('center_axis',(0.86081688607418,-0.5,0.0948382235680992));
#19739=DIRECTION('ref_axis',(0.109509747813016,-1.37062880361661E-18,-0.993985721795806));
#19740=DIRECTION('',(-0.109509747813016,1.50231459873716E-16,0.993985721795806));
#19741=DIRECTION('',(0.496992860897903,0.866025403784439,0.054754873906508));
#19742=DIRECTION('',(0.109509747813016,-3.00462919747432E-16,-0.993985721795806));
#19743=DIRECTION('center_axis',(0.496992860897903,0.866025403784439,0.0547548739065076));
#19744=DIRECTION('ref_axis',(0.109509747813015,-2.68836199388207E-18,-0.993985721795806));
#19745=DIRECTION('center_axis',(0.496992860897903,0.866025403784439,0.0547548739065076));
#19746=DIRECTION('ref_axis',(-0.86081688607418,0.5,-0.0948382235681014));
#19747=DIRECTION('',(0.86081688607418,-0.5,0.0948382235680992));
#19748=DIRECTION('',(-0.109509747813016,0.,0.993985721795806));
#19749=DIRECTION('',(0.86081688607418,-0.5,0.0948382235680992));
#19750=DIRECTION('center_axis',(-0.86081688607418,0.5,-0.0948382235680992));
#19751=DIRECTION('ref_axis',(-0.109509747813016,1.37062880361661E-18,0.993985721795806));
#19752=DIRECTION('',(0.496992860897903,0.866025403784439,0.0547548739065076));
#19753=DIRECTION('',(0.109509747813016,3.12982208070242E-16,-0.993985721795806));
#19754=DIRECTION('',(-0.496992860897903,-0.866025403784439,-0.0547548739065082));
#19755=DIRECTION('center_axis',(0.109509747813016,0.,-0.993985721795806));
#19756=DIRECTION('ref_axis',(0.,-1.,0.));
#19757=DIRECTION('',(0.86081688607418,-0.5,0.0948382235680992));
#19758=DIRECTION('center_axis',(-0.496992860897903,-0.866025403784439,-0.0547548739065078));
#19759=DIRECTION('ref_axis',(-0.86081688607418,0.5,-0.0948382235680992));
#19760=DIRECTION('center_axis',(-0.496992860897903,-0.866025403784439,-0.0547548739065078));
#19761=DIRECTION('ref_axis',(0.86081688607418,-0.5,0.0948382235681014));
#19762=DIRECTION('',(0.86081688607418,-0.5,0.0948382235680992));
#19763=DIRECTION('center_axis',(-0.109509747813016,0.,0.993985721795806));
#19764=DIRECTION('ref_axis',(0.993985721795806,0.,0.109509747813016));
#19765=DIRECTION('center_axis',(0.496992860897903,0.866025403784439,0.054754873906508));
#19766=DIRECTION('ref_axis',(0.86081688607418,-0.5,0.0948382235681014));
#19767=DIRECTION('center_axis',(-0.993985721795806,6.12303176911189E-17,
-0.109509747813016));
#19768=DIRECTION('ref_axis',(-0.109509747813016,-4.27307853354592E-34,0.993985721795806));
#19769=DIRECTION('',(-3.7115920228551E-17,-1.,-2.22241612446982E-16));
#19770=DIRECTION('',(1.08354344120878E-16,1.,-4.24367274947369E-16));
#19771=DIRECTION('center_axis',(-0.496992860897903,-0.866025403784439,-0.054754873906508));
#19772=DIRECTION('ref_axis',(-0.86081688607418,0.5,-0.0948382235680945));
#19773=DIRECTION('center_axis',(-0.496992860897903,-0.866025403784439,-0.0547548739065078));
#19774=DIRECTION('ref_axis',(0.86081688607418,-0.5,0.0948382235680946));
#19775=DIRECTION('',(-0.496992860897903,-0.866025403784439,-0.054754873906508));
#19776=DIRECTION('center_axis',(0.496992860897903,0.866025403784439,0.0547548739065076));
#19777=DIRECTION('ref_axis',(-0.86081688607418,0.5,-0.0948382235680945));
#19778=DIRECTION('',(0.496992860897903,0.866025403784439,0.054754873906508));
#19779=DIRECTION('center_axis',(0.86081688607418,-0.5,0.0948382235680992));
#19780=DIRECTION('ref_axis',(0.109509747813016,-1.37062880361661E-18,-0.993985721795806));
#19781=DIRECTION('',(-0.109509747813016,1.50231459873716E-16,0.993985721795806));
#19782=DIRECTION('',(0.496992860897903,0.866025403784439,0.054754873906508));
#19783=DIRECTION('',(0.109509747813016,-3.00462919747432E-16,-0.993985721795806));
#19784=DIRECTION('center_axis',(0.496992860897903,0.866025403784439,0.0547548739065076));
#19785=DIRECTION('ref_axis',(0.109509747813015,-2.68836199388207E-18,-0.993985721795806));
#19786=DIRECTION('center_axis',(0.496992860897903,0.866025403784439,0.0547548739065076));
#19787=DIRECTION('ref_axis',(-0.86081688607418,0.5,-0.0948382235680945));
#19788=DIRECTION('',(-0.86081688607418,0.5,-0.0948382235680992));
#19789=DIRECTION('',(0.86081688607418,-0.5,0.0948382235680992));
#19790=DIRECTION('',(-0.109509747813016,0.,0.993985721795806));
#19791=DIRECTION('',(0.86081688607418,-0.5,0.0948382235680992));
#19792=DIRECTION('',(-0.86081688607418,0.5,-0.0948382235680992));
#19793=DIRECTION('center_axis',(-0.86081688607418,0.5,-0.0948382235680992));
#19794=DIRECTION('ref_axis',(-0.109509747813016,1.37062880361661E-18,0.993985721795806));
#19795=DIRECTION('',(0.496992860897903,0.866025403784439,0.0547548739065076));
#19796=DIRECTION('',(0.109509747813016,3.12982208070242E-16,-0.993985721795806));
#19797=DIRECTION('',(-0.496992860897903,-0.866025403784439,-0.0547548739065082));
#19798=DIRECTION('center_axis',(0.109509747813016,0.,-0.993985721795806));
#19799=DIRECTION('ref_axis',(0.,-1.,0.));
#19800=DIRECTION('',(0.86081688607418,-0.5,0.0948382235680992));
#19801=DIRECTION('center_axis',(-0.496992860897903,-0.866025403784439,-0.0547548739065078));
#19802=DIRECTION('ref_axis',(-0.86081688607418,0.5,-0.0948382235680992));
#19803=DIRECTION('',(-0.86081688607418,0.5,-0.0948382235680992));
#19804=DIRECTION('center_axis',(-0.496992860897903,-0.866025403784439,-0.0547548739065078));
#19805=DIRECTION('ref_axis',(0.86081688607418,-0.5,0.0948382235680946));
#19806=DIRECTION('',(-0.86081688607418,0.5,-0.0948382235680992));
#19807=DIRECTION('',(0.86081688607418,-0.5,0.0948382235680992));
#19808=DIRECTION('center_axis',(0.109509747813016,0.,-0.993985721795806));
#19809=DIRECTION('ref_axis',(0.,-1.,0.));
#19810=DIRECTION('',(-0.496992860897903,-0.866025403784439,-0.054754873906508));
#19811=DIRECTION('',(0.756106594798299,-0.64912524734226,0.0833020441848256));
#19812=DIRECTION('center_axis',(-0.109509747813016,0.,0.993985721795806));
#19813=DIRECTION('ref_axis',(0.993985721795806,0.,0.109509747813016));
#19814=DIRECTION('',(-0.756106594798299,0.64912524734226,-0.0833020441848256));
#19815=DIRECTION('center_axis',(-0.109509747813016,0.,0.993985721795806));
#19816=DIRECTION('ref_axis',(0.993985721795806,0.,0.109509747813016));
#19817=DIRECTION('center_axis',(0.496992860897903,0.866025403784439,0.054754873906508));
#19818=DIRECTION('ref_axis',(0.86081688607418,-0.5,0.0948382235680945));
#19819=DIRECTION('center_axis',(0.645221227515378,0.760681545236145,0.0710855421355126));
#19820=DIRECTION('ref_axis',(0.109509747813016,-3.16883939248426E-18,-0.993985721795806));
#19821=DIRECTION('',(-0.756106594798299,0.64912524734226,-0.0833020441848257));
#19822=DIRECTION('',(0.756106594798299,-0.64912524734226,0.0833020441848256));
#19823=DIRECTION('center_axis',(-0.645221227515378,-0.760681545236145,-0.0710855421355126));
#19824=DIRECTION('ref_axis',(-0.756106594798299,0.64912524734226,-0.0833020441848256));
#19825=DIRECTION('',(-0.756106594798299,0.64912524734226,-0.0833020441848256));
#19826=DIRECTION('',(0.756106594798299,-0.64912524734226,0.0833020441848256));
#19827=DIRECTION('center_axis',(-0.496992860897903,0.866025403784439,-0.054754873906508));
#19828=DIRECTION('ref_axis',(0.86081688607418,0.5,0.0948382235680945));
#19829=DIRECTION('center_axis',(-0.496992860897903,0.866025403784439,-0.0547548739065078));
#19830=DIRECTION('ref_axis',(-0.86081688607418,-0.5,-0.0948382235680946));
#19831=DIRECTION('',(-0.496992860897903,0.866025403784439,-0.054754873906508));
#19832=DIRECTION('center_axis',(0.496992860897903,-0.866025403784439,0.0547548739065076));
#19833=DIRECTION('ref_axis',(0.86081688607418,0.5,0.0948382235680945));
#19834=DIRECTION('',(0.496992860897903,-0.866025403784439,0.054754873906508));
#19835=DIRECTION('center_axis',(0.109509747813016,0.,-0.993985721795806));
#19836=DIRECTION('ref_axis',(0.,-1.,0.));
#19837=DIRECTION('',(0.756106594798299,-0.64912524734226,0.0833020441848256));
#19838=DIRECTION('',(-0.86081688607418,-0.5,-0.0948382235680992));
#19839=DIRECTION('',(-0.86081688607418,-0.5,-0.0948382235680992));
#19840=DIRECTION('center_axis',(-0.496992860897903,0.866025403784439,-0.0547548739065078));
#19841=DIRECTION('ref_axis',(-0.109509747813016,-8.62567737696967E-18,0.993985721795806));
#19842=DIRECTION('',(-0.109509747813016,-1.50231459873716E-16,0.993985721795806));
#19843=DIRECTION('center_axis',(-0.496992860897903,0.866025403784439,-0.0547548739065078));
#19844=DIRECTION('ref_axis',(-0.86081688607418,-0.5,-0.0948382235680946));
#19845=DIRECTION('',(-0.86081688607418,-0.5,-0.0948382235680992));
#19846=DIRECTION('center_axis',(-0.756106594798299,0.64912524734226,-0.0833020441848257));
#19847=DIRECTION('ref_axis',(0.645221227515378,0.760681545236146,0.0710855421355019));
#19848=DIRECTION('center_axis',(0.496992860897903,-0.866025403784439,0.054754873906508));
#19849=DIRECTION('ref_axis',(-0.86081688607418,-0.5,-0.0948382235680945));
#19850=DIRECTION('',(-0.496992860897903,0.866025403784439,-0.054754873906508));
#19851=DIRECTION('center_axis',(0.496992860897903,-0.866025403784439,0.0547548739065076));
#19852=DIRECTION('ref_axis',(0.86081688607418,0.5,0.0948382235680945));
#19853=DIRECTION('',(0.496992860897903,-0.866025403784439,0.054754873906508));
#19854=DIRECTION('center_axis',(-0.756106594798299,0.64912524734226,-0.0833020441848257));
#19855=DIRECTION('ref_axis',(0.645221227515378,0.760681545236146,0.0710855421355018));
#19856=DIRECTION('',(-0.756106594798299,0.64912524734226,-0.0833020441848256));
#19857=DIRECTION('center_axis',(0.756106594798299,-0.64912524734226,0.0833020441848257));
#19858=DIRECTION('ref_axis',(-0.645221227515378,-0.760681545236146,-0.0710855421355019));
#19859=DIRECTION('center_axis',(0.496992860897903,-0.866025403784439,0.0547548739065076));
#19860=DIRECTION('ref_axis',(0.109509747813016,4.04398041928102E-16,-0.993985721795806));
#19861=DIRECTION('',(-0.86081688607418,-0.5,-0.0948382235680992));
#19862=DIRECTION('',(0.109509747813016,3.00462919747432E-16,-0.993985721795806));
#19863=DIRECTION('center_axis',(0.109509747813016,0.,-0.993985721795806));
#19864=DIRECTION('ref_axis',(0.,-1.,0.));
#19865=DIRECTION('center_axis',(-0.756106594798299,0.64912524734226,-0.0833020441848257));
#19866=DIRECTION('ref_axis',(0.645221227515378,0.760681545236146,0.0710855421355019));
#19867=DIRECTION('center_axis',(-0.86081688607418,-0.5,-0.0948382235680992));
#19868=DIRECTION('ref_axis',(-0.496992860897903,0.866025403784439,-0.054754873906508));
#19869=DIRECTION('center_axis',(-0.109509747813016,0.,0.993985721795806));
#19870=DIRECTION('ref_axis',(0.993985721795806,0.,0.109509747813016));
#19871=DIRECTION('center_axis',(-0.109509747813016,0.,0.993985721795806));
#19872=DIRECTION('ref_axis',(0.993985721795806,0.,0.109509747813016));
#19873=DIRECTION('center_axis',(0.109509747813016,0.,-0.993985721795806));
#19874=DIRECTION('ref_axis',(0.,-1.,0.));
#19875=DIRECTION('center_axis',(0.109509747813016,0.,-0.993985721795806));
#19876=DIRECTION('ref_axis',(0.,-1.,0.));
#19877=DIRECTION('center_axis',(0.,1.,0.));
#19878=DIRECTION('ref_axis',(0.993985721795806,0.,0.109509747813016));
#19879=DIRECTION('',(-0.993985721795806,0.,-0.109509747813016));
#19880=DIRECTION('',(-0.109509747813016,0.,0.993985721795806));
#19881=DIRECTION('',(-0.993985721795806,0.,-0.109509747813016));
#19882=DIRECTION('',(-0.109509747813016,0.,0.993985721795806));
#19883=DIRECTION('center_axis',(0.993985721795806,0.,0.109509747813016));
#19884=DIRECTION('ref_axis',(0.,1.,0.));
#19885=DIRECTION('',(0.,1.,0.));
#19886=DIRECTION('',(-0.109509747813016,0.,0.993985721795806));
#19887=DIRECTION('',(0.,1.,0.));
#19888=DIRECTION('center_axis',(-0.993985721795806,0.,-0.109509747813016));
#19889=DIRECTION('ref_axis',(-0.109509747813016,0.,0.993985721795806));
#19890=DIRECTION('',(0.,1.,0.));
#19891=DIRECTION('',(-0.109509747813016,0.,0.993985721795806));
#19892=DIRECTION('',(0.,1.,0.));
#19893=DIRECTION('',(0.109509747813016,0.,-0.993985721795806));
#19894=DIRECTION('center_axis',(-0.109509747813016,0.,0.993985721795806));
#19895=DIRECTION('ref_axis',(-0.993985721795806,0.,-0.109509747813016));
#19896=DIRECTION('center_axis',(-0.109509747813016,0.,0.993985721795806));
#19897=DIRECTION('ref_axis',(0.993985721795806,0.,0.109509747813016));
#19898=DIRECTION('',(-0.109509747813016,0.,0.993985721795806));
#19899=DIRECTION('center_axis',(0.109509747813016,0.,-0.993985721795806));
#19900=DIRECTION('ref_axis',(0.993985721795806,0.,0.109509747813016));
#19901=DIRECTION('center_axis',(0.,1.,0.));
#19902=DIRECTION('ref_axis',(0.993985721795806,0.,0.109509747813016));
#19903=DIRECTION('',(0.993985721795806,0.,0.109509747813016));
#19904=DIRECTION('',(0.109509747813016,0.,-0.993985721795806));
#19905=DIRECTION('',(0.993985721795806,0.,0.109509747813016));
#19906=DIRECTION('center_axis',(-0.109509747813016,0.,0.993985721795806));
#19907=DIRECTION('ref_axis',(-0.993985721795806,0.,-0.109509747813016));
#19908=DIRECTION('center_axis',(-0.109509747813016,0.,0.993985721795806));
#19909=DIRECTION('ref_axis',(0.993985721795806,0.,0.109509747813016));
#19910=DIRECTION('',(-0.109509747813016,0.,0.993985721795806));
#19911=DIRECTION('center_axis',(0.109509747813016,0.,-0.993985721795806));
#19912=DIRECTION('ref_axis',(0.993985721795806,0.,0.109509747813016));
#19913=DIRECTION('center_axis',(0.993985721795806,0.,0.109509747813016));
#19914=DIRECTION('ref_axis',(0.,1.,0.));
#19915=DIRECTION('',(0.,-1.,0.));
#19916=DIRECTION('',(0.,-1.,0.));
#19917=DIRECTION('',(0.109509747813016,0.,-0.993985721795806));
#19918=DIRECTION('center_axis',(-0.109509747813016,0.,0.993985721795806));
#19919=DIRECTION('ref_axis',(0.993985721795806,0.,0.109509747813016));
#19920=DIRECTION('center_axis',(-0.109509747813016,0.,0.993985721795806));
#19921=DIRECTION('ref_axis',(0.993985721795806,0.,0.109509747813016));
#19922=DIRECTION('',(-0.993985721795806,0.,-0.109509747813016));
#19923=DIRECTION('center_axis',(-0.109509747813016,0.,0.993985721795806));
#19924=DIRECTION('ref_axis',(0.993985721795806,0.,0.109509747813016));
#19925=DIRECTION('center_axis',(-0.109509747813016,0.,0.993985721795806));
#19926=DIRECTION('ref_axis',(-0.993985721795806,0.,-0.109509747813016));
#19927=DIRECTION('',(-0.109509747813016,0.,0.993985721795806));
#19928=DIRECTION('center_axis',(0.109509747813016,0.,-0.993985721795806));
#19929=DIRECTION('ref_axis',(0.993985721795806,0.,0.109509747813016));
#19930=DIRECTION('center_axis',(-0.109509747813016,0.,0.993985721795806));
#19931=DIRECTION('ref_axis',(0.993985721795806,0.,0.109509747813016));
#19932=DIRECTION('',(-0.993985721795806,0.,-0.109509747813016));
#19933=DIRECTION('center_axis',(0.109509747813016,0.,-0.993985721795806));
#19934=DIRECTION('ref_axis',(0.993985721795806,0.,0.109509747813016));
#19935=DIRECTION('',(0.993985721795806,0.,0.109509747813016));
#19936=DIRECTION('',(0.,-1.,0.));
#19937=DIRECTION('center_axis',(0.,-1.,0.));
#19938=DIRECTION('ref_axis',(0.109509747813016,0.,-0.993985721795806));
#19939=DIRECTION('',(0.109509747813016,0.,-0.993985721795806));
#19940=DIRECTION('center_axis',(0.,-1.,0.));
#19941=DIRECTION('ref_axis',(0.109509747813016,0.,-0.993985721795806));
#19942=DIRECTION('',(-0.109509747813016,0.,0.993985721795806));
#19943=DIRECTION('',(0.993985721795806,0.,0.109509747813016));
#19944=DIRECTION('center_axis',(0.109509747813016,0.,-0.993985721795806));
#19945=DIRECTION('ref_axis',(0.,-1.,0.));
#19946=DIRECTION('',(0.,-1.,0.));
#19947=DIRECTION('center_axis',(-0.993985721795806,0.,-0.109509747813016));
#19948=DIRECTION('ref_axis',(-0.109509747813016,0.,0.993985721795806));
#19949=DIRECTION('center_axis',(-0.109509747813016,0.,0.993985721795806));
#19950=DIRECTION('ref_axis',(-0.993985721795806,0.,-0.109509747813016));
#44531=CARTESIAN_POINT('',(0.,0.,0.));
#44532=CARTESIAN_POINT('Origin',(-12.6095156787167,81.500000021449,118.014000374155));
#44533=CARTESIAN_POINT('',(2.32160098384069,81.500000021449,23.5811578282542));
#44534=CARTESIAN_POINT('',(2.3435029334033,81.500000021449,23.3823606838951));
#44535=CARTESIAN_POINT('',(-8.13657993063557,81.500000021449,118.506794239313));
#44536=CARTESIAN_POINT('',(1.55268733299948,78.977364418784,23.4964448005445));
#44537=CARTESIAN_POINT('Origin',(-2.15133476424044,81.5,23.0883639630957));
#44538=CARTESIAN_POINT('',(1.30589978067932,78.5789363917495,22.9662303004148));
#44539=CARTESIAN_POINT('Ctrl Pts',(1.55268732841254,78.9773644228491,23.4964448000391));
#44540=CARTESIAN_POINT('Ctrl Pts',(1.51761375586145,78.9252402998144,23.4925806618552));
#44541=CARTESIAN_POINT('Ctrl Pts',(1.48036107708696,78.8704476794957,23.4759347437579));
#44542=CARTESIAN_POINT('Ctrl Pts',(1.41282928245068,78.7711847504358,23.4172138237909));
#44543=CARTESIAN_POINT('Ctrl Pts',(1.38261235100385,78.7266711800993,23.3751404616741));
#44544=CARTESIAN_POINT('Ctrl Pts',(1.33718570603301,78.657182012345,23.2807163565727));
#44545=CARTESIAN_POINT('Ctrl Pts',(1.31893775138881,78.6275451314688,23.2221451156177));
#44546=CARTESIAN_POINT('Ctrl Pts',(1.29982863988694,78.5884467386214,23.0961031394044));
#44547=CARTESIAN_POINT('Ctrl Pts',(1.29902406364269,78.5789363962849,23.0286389844206));
#44548=CARTESIAN_POINT('Ctrl Pts',(1.30589977539658,78.5789363962849,22.9662302998328));
#44549=CARTESIAN_POINT('',(1.36065465458583,78.5789363917495,22.4692374395169));
#44550=CARTESIAN_POINT('',(0.867860795006342,78.5789363869598,26.9421731882127));
#44551=CARTESIAN_POINT('',(1.07173072593556,78.2166828749042,21.9343806755756));
#44552=CARTESIAN_POINT('Ctrl Pts',(1.36065464930308,78.5789363962848,22.4692374389349));
#44553=CARTESIAN_POINT('Ctrl Pts',(1.36753036105647,78.5789363962848,22.4068287543516));
#44554=CARTESIAN_POINT('Ctrl Pts',(1.3668087207202,78.5693548526245,22.3393737366166));
#44555=CARTESIAN_POINT('Ctrl Pts',(1.34704682518434,78.5308168815584,22.2132598416578));
#44556=CARTESIAN_POINT('Ctrl Pts',(1.32794969506718,78.5019090265213,22.154595045046));
#44557=CARTESIAN_POINT('Ctrl Pts',(1.2781466042549,78.4361770822946,22.0596887765826));
#44558=CARTESIAN_POINT('Ctrl Pts',(1.24408431979824,78.3949647868373,22.0171917628595));
#44559=CARTESIAN_POINT('Ctrl Pts',(1.16372704304608,78.3067126653714,21.9570578293212));
#44560=CARTESIAN_POINT('Ctrl Pts',(1.1173804610504,78.2597272540181,21.9394100143986));
#44561=CARTESIAN_POINT('Ctrl Pts',(1.07173071992196,78.2166828799263,21.934380674913));
#44562=CARTESIAN_POINT('',(2.48586560556021,81.500000021449,22.0901792455605));
#44563=CARTESIAN_POINT('Origin',(-1.98707014252092,81.5,21.597385380402));
#44564=CARTESIAN_POINT('',(2.81439485066613,81.500000021449,19.1082220597325));
#44565=CARTESIAN_POINT('',(-8.13657993063557,81.500000021449,118.506794239313));
#44566=CARTESIAN_POINT('Origin',(-1.658540897415,81.500000021449,18.615428194574));
#44567=CARTESIAN_POINT('',(2.22867057917708,79.9960688658798,22.061843463808));
#44568=CARTESIAN_POINT('Origin',(-1.98707014252092,81.5,21.597385380402));
#44569=CARTESIAN_POINT('',(2.08630790702017,79.9960688658798,23.3540249021425));
#44570=CARTESIAN_POINT('',(1.681121840112,79.9960688658798,27.031772072787));
#44571=CARTESIAN_POINT('Origin',(-2.12943281467784,81.5,22.8895668187365));
#44572=CARTESIAN_POINT('Origin',(-12.6095156787167,81.500000021449,118.014000374155));
#44573=CARTESIAN_POINT('',(2.08067953865206,81.500000021449,25.767926416205));
#44574=CARTESIAN_POINT('',(2.10258148821465,81.500000021449,25.5691292718459));
#44575=CARTESIAN_POINT('',(-8.13657993063557,81.500000021449,118.506794239313));
#44576=CARTESIAN_POINT('',(1.84538646183153,83.0039311341202,25.5407934900933));
#44577=CARTESIAN_POINT('Origin',(-2.37035425986648,81.5,25.0763354066873));
#44578=CARTESIAN_POINT('',(2.06440595745756,83.0039311341202,23.5528220465017));
#44579=CARTESIAN_POINT('',(1.681121840112,83.0039311341202,27.031772072787));
#44580=CARTESIAN_POINT('Origin',(-2.15133476424044,81.5,23.0883639630957));
#44581=CARTESIAN_POINT('',(-2.12943281467784,86.0000000007247,22.8895668187365));
#44582=CARTESIAN_POINT('Origin',(-2.12943281467784,81.5,22.8895668187365));
#44583=CARTESIAN_POINT('',(-2.39225620942908,86.0000000007247,25.2751325510465));
#44584=CARTESIAN_POINT('',(-2.12943281467784,86.,22.8895668187365));
#44585=CARTESIAN_POINT('Origin',(-2.39225620942908,81.5,25.2751325510465));
#44586=CARTESIAN_POINT('Origin',(-12.6095156787167,81.500000021449,118.014000374155));
#44587=CARTESIAN_POINT('',(-7.31525682145931,81.500000021449,111.051901325908));
#44588=CARTESIAN_POINT('',(-7.2933548718967,81.500000021449,110.853104181549));
#44589=CARTESIAN_POINT('',(-8.13657993063557,81.500000021449,118.506794239313));
#44590=CARTESIAN_POINT('',(-8.0841704721213,78.9773644192325,110.967188298218));
#44591=CARTESIAN_POINT('Origin',(-11.7881925695404,81.5,110.55910746075));
#44592=CARTESIAN_POINT('',(-8.33095802467381,78.5789363917952,110.436973798063));
#44593=CARTESIAN_POINT('Ctrl Pts',(-8.0841704768878,78.9773644228493,110.967188297693));
#44594=CARTESIAN_POINT('Ctrl Pts',(-8.11924404944169,78.9252402998083,110.963324159568));
#44595=CARTESIAN_POINT('Ctrl Pts',(-8.15649672821697,78.8704476794907,110.94667824141));
#44596=CARTESIAN_POINT('Ctrl Pts',(-8.22402852285583,78.7711847504269,110.887957321438));
#44597=CARTESIAN_POINT('Ctrl Pts',(-8.25424545430345,78.7266711800892,110.845883959318));
#44598=CARTESIAN_POINT('Ctrl Pts',(-8.29967209927197,78.6571820123377,110.751459854213));
#44599=CARTESIAN_POINT('Ctrl Pts',(-8.31792005391415,78.6275451314643,110.69288861326));
#44600=CARTESIAN_POINT('Ctrl Pts',(-8.33702916541348,78.5884467386206,110.566846637052));
#44601=CARTESIAN_POINT('Ctrl Pts',(-8.33783374165725,78.5789363962851,110.499382482071));
#44602=CARTESIAN_POINT('Ctrl Pts',(-8.33095802990372,78.5789363962851,110.436973797487));
#44603=CARTESIAN_POINT('',(-8.27620315076731,78.5789363917951,109.939980937165));
#44604=CARTESIAN_POINT('',(-8.76899701029366,78.5789363869598,114.412916685867));
#44605=CARTESIAN_POINT('',(-8.56512707942982,78.2166828749152,109.405124173222));
#44606=CARTESIAN_POINT('Ctrl Pts',(-8.27620315599722,78.5789363962851,109.939980936589));
#44607=CARTESIAN_POINT('Ctrl Pts',(-8.26932744424383,78.5789363962851,109.877572252006));
#44608=CARTESIAN_POINT('Ctrl Pts',(-8.2700490845801,78.5693548526248,109.810117234271));
#44609=CARTESIAN_POINT('Ctrl Pts',(-8.28981098011595,78.5308168815586,109.684003339312));
#44610=CARTESIAN_POINT('Ctrl Pts',(-8.30890811023311,78.5019090265215,109.6253385427));
#44611=CARTESIAN_POINT('Ctrl Pts',(-8.35871120104538,78.4361770822949,109.530432274237));
#44612=CARTESIAN_POINT('Ctrl Pts',(-8.39277348550203,78.3949647868375,109.487935260513));
#44613=CARTESIAN_POINT('Ctrl Pts',(-8.47313076225417,78.3067126653716,109.427801326975));
#44614=CARTESIAN_POINT('Ctrl Pts',(-8.51947734424986,78.2597272540184,109.410153512053));
#44615=CARTESIAN_POINT('Ctrl Pts',(-8.56512708537829,78.2166828799266,109.405124172567));
#44616=CARTESIAN_POINT('',(-7.15099219973979,81.500000021449,109.560922743215));
#44617=CARTESIAN_POINT('Origin',(-11.6239279478209,81.5,109.068128878056));
#44618=CARTESIAN_POINT('',(1.93831686649513,81.500000021449,27.0601078545396));
#44619=CARTESIAN_POINT('',(-8.13657993063557,81.500000021449,118.506794239313));
#44620=CARTESIAN_POINT('',(0.524181986870476,78.2166828749042,26.9043092845546));
#44621=CARTESIAN_POINT('Origin',(-2.534618881586,81.5,26.567313989381));
#44622=CARTESIAN_POINT('',(0.922615663333761,78.5789363917495,26.4451803267001));
#44623=CARTESIAN_POINT('Ctrl Pts',(0.524181980856895,78.2166828799263,26.9043092838921));
#44624=CARTESIAN_POINT('Ctrl Pts',(0.569831721989357,78.2597272540282,26.9093386232555));
#44625=CARTESIAN_POINT('Ctrl Pts',(0.618908660925751,78.3067126653714,26.9022038424795));
#44626=CARTESIAN_POINT('Ctrl Pts',(0.71042987961836,78.3949647868373,26.8610061675593));
#44627=CARTESIAN_POINT('Ctrl Pts',(0.752926883593083,78.4361770822946,26.8269438709403));
#44628=CARTESIAN_POINT('Ctrl Pts',(0.822196767061209,78.5019090265213,26.7451561524711));
#44629=CARTESIAN_POINT('Ctrl Pts',(0.853607315213045,78.5308168815584,26.69205590572));
#44630=CARTESIAN_POINT('Ctrl Pts',(0.900350505106304,78.5693548526245,26.5732690326429));
#44631=CARTESIAN_POINT('Ctrl Pts',(0.915739946297612,78.5789363962848,26.5075890107014));
#44632=CARTESIAN_POINT('Ctrl Pts',(0.922615658051007,78.5789363962848,26.4451803261182));
#44633=CARTESIAN_POINT('',(0.977370537240269,78.5789363917495,25.9481874658022));
#44634=CARTESIAN_POINT('',(0.867860795006342,78.5789363869598,26.9421731882127));
#44635=CARTESIAN_POINT('',(1.33366783737344,78.977364418784,25.4844162441361));
#44636=CARTESIAN_POINT('Ctrl Pts',(0.977370531957515,78.5789363962848,25.9481874652202));
#44637=CARTESIAN_POINT('Ctrl Pts',(0.984246243711048,78.5789363962848,25.8857787806357));
#44638=CARTESIAN_POINT('Ctrl Pts',(0.999718620810108,78.5884467386204,25.8201078959373));
#44639=CARTESIAN_POINT('Ctrl Pts',(1.04580902666772,78.627545131464,25.7012491041017));
#44640=CARTESIAN_POINT('Ctrl Pts',(1.07637039934524,78.6571820123375,25.6480553016858));
#44641=CARTESIAN_POINT('Ctrl Pts',(1.14126383696667,78.726671180089,25.5657854198846));
#44642=CARTESIAN_POINT('Ctrl Pts',(1.17991548793108,78.7711847504267,25.5312994716744));
#44643=CARTESIAN_POINT('Ctrl Pts',(1.25861122451092,78.8704476794904,25.4886887831835));
#44644=CARTESIAN_POINT('Ctrl Pts',(1.29859426023195,78.9252402998056,25.4805521055439));
#44645=CARTESIAN_POINT('Ctrl Pts',(1.33366783278649,78.977364422849,25.4844162436308));
#44646=CARTESIAN_POINT('Origin',(-2.37035425986648,81.5,25.0763354066873));
#44647=CARTESIAN_POINT('',(1.82348451226893,79.9960688658798,25.7395906344525));
#44648=CARTESIAN_POINT('Origin',(-2.39225620942908,81.5,25.2751325510465));
#44649=CARTESIAN_POINT('',(1.681121840112,79.9960688658798,27.031772072787));
#44650=CARTESIAN_POINT('',(1.681121840112,79.9960688658798,27.031772072787));
#44651=CARTESIAN_POINT('Origin',(-2.534618881586,81.5,26.567313989381));
#44652=CARTESIAN_POINT('',(-7.40818722558546,79.9960688674047,109.532586961521));
#44653=CARTESIAN_POINT('Origin',(-11.6239279478209,81.5,109.068128878056));
#44654=CARTESIAN_POINT('',(-7.55054989827983,79.9960688658798,110.824768399797));
#44655=CARTESIAN_POINT('',(-7.955735965188,79.9960688658798,114.502515570441));
#44656=CARTESIAN_POINT('Origin',(-11.7662906199778,81.5,110.360310316391));
#44657=CARTESIAN_POINT('Origin',(-12.6095156787167,81.500000021449,118.014000374155));
#44658=CARTESIAN_POINT('',(-8.13657993063557,81.500000021449,118.506794239313));
#44659=CARTESIAN_POINT('Origin',(-12.6095156787167,81.500000021449,118.014000374155));
#44660=CARTESIAN_POINT('',(-7.69854093880487,81.500000021449,114.530851352194));
#44661=CARTESIAN_POINT('',(-8.13657993063557,81.500000021449,118.506794239313));
#44662=CARTESIAN_POINT('',(-9.11267581892563,78.2166828745796,114.375052782154));
#44663=CARTESIAN_POINT('Origin',(-12.171476686886,81.5,114.038057487035));
#44664=CARTESIAN_POINT('',(-8.71424214201937,78.5789363917952,113.915923824348));
#44665=CARTESIAN_POINT('Ctrl Pts',(-9.11267582444339,78.2166828799266,114.375052781546));
#44666=CARTESIAN_POINT('Ctrl Pts',(-9.06702608331569,78.2597272540202,114.380082120982));
#44667=CARTESIAN_POINT('Ctrl Pts',(-9.01794914437927,78.3067126653671,114.372947340134));
#44668=CARTESIAN_POINT('Ctrl Pts',(-8.92642792569046,78.3949647868293,114.331749665219));
#44669=CARTESIAN_POINT('Ctrl Pts',(-8.88393092171716,78.4361770822852,114.297687368603));
#44670=CARTESIAN_POINT('Ctrl Pts',(-8.81466103824691,78.5019090265143,114.215899650137));
#44671=CARTESIAN_POINT('Ctrl Pts',(-8.78325049009251,78.530816881554,114.162799403385));
#44672=CARTESIAN_POINT('Ctrl Pts',(-8.73650730019552,78.5693548526238,114.044012530303));
#44673=CARTESIAN_POINT('Ctrl Pts',(-8.72111785900304,78.5789363962851,113.978332508359));
#44674=CARTESIAN_POINT('Ctrl Pts',(-8.71424214724929,78.5789363962851,113.915923823772));
#44675=CARTESIAN_POINT('',(-8.65948726811286,78.5789363917952,113.41893096345));
#44676=CARTESIAN_POINT('',(-8.76899701029366,78.5789363869598,114.412916685867));
#44677=CARTESIAN_POINT('',(-8.30318996795119,78.9773644188579,112.955159741787));
#44678=CARTESIAN_POINT('Ctrl Pts',(-8.65948727334278,78.5789363962851,113.418930962874));
#44679=CARTESIAN_POINT('Ctrl Pts',(-8.65261156158889,78.5789363962851,113.356522278286));
#44680=CARTESIAN_POINT('Ctrl Pts',(-8.63713918448864,78.5884467386216,113.290851393585));
#44681=CARTESIAN_POINT('Ctrl Pts',(-8.59104877862742,78.627545131469,113.171992601745));
#44682=CARTESIAN_POINT('Ctrl Pts',(-8.5604874059475,78.6571820123452,113.118798799327));
#44683=CARTESIAN_POINT('Ctrl Pts',(-8.49559396832452,78.7266711800996,113.03652891753));
#44684=CARTESIAN_POINT('Ctrl Pts',(-8.45694231736169,78.771184750436,113.002042969323));
#44685=CARTESIAN_POINT('Ctrl Pts',(-8.37824658078551,78.870447679496,112.959432280837));
#44686=CARTESIAN_POINT('Ctrl Pts',(-8.33826354506655,78.9252402998085,112.951295603198));
#44687=CARTESIAN_POINT('Ctrl Pts',(-8.30318997251383,78.9773644228493,112.955159741285));
#44688=CARTESIAN_POINT('',(-7.53427631708535,81.500000021449,113.0398727695));
#44689=CARTESIAN_POINT('Origin',(-12.0072120651665,81.5,112.547078904341));
#44690=CARTESIAN_POINT('',(-7.55617826664794,81.500000021449,113.238669913859));
#44691=CARTESIAN_POINT('',(-8.13657993063557,81.500000021449,118.506794239313));
#44692=CARTESIAN_POINT('',(-7.81337329303107,79.9960688658798,113.210334132106));
#44693=CARTESIAN_POINT('Origin',(-12.0291140147291,81.5,112.7458760487));
#44694=CARTESIAN_POINT('',(-7.95573596518799,79.9960688658798,114.502515570441));
#44695=CARTESIAN_POINT('',(-7.955735965188,79.9960688658798,114.502515570441));
#44696=CARTESIAN_POINT('Origin',(-12.171476686886,81.5,114.038057487035));
#44697=CARTESIAN_POINT('Origin',(-2.534618881586,81.5,26.567313989381));
#44698=CARTESIAN_POINT('',(-7.45399161239785,81.5,20.9950817674304));
#44699=CARTESIAN_POINT('',(-8.00154035146294,81.5,25.9650103764094));
#44700=CARTESIAN_POINT('',(-8.00154035146294,81.5,25.9650103764094));
#44701=CARTESIAN_POINT('',(1.83168562221586,77.5642538212272,22.0181066961974));
#44702=CARTESIAN_POINT('Origin',(-1.98707014252092,81.5,21.597385380402));
#44703=CARTESIAN_POINT('',(2.11676125496322,77.9298111396176,22.5525394843164));
#44704=CARTESIAN_POINT('Ctrl Pts',(1.83168562221586,77.5642538212272,22.0181066961974));
#44705=CARTESIAN_POINT('Ctrl Pts',(1.87641861446953,77.6081839481971,22.0230350353005));
#44706=CARTESIAN_POINT('Ctrl Pts',(1.9219453311641,77.6558998044383,22.0406193987957));
#44707=CARTESIAN_POINT('Ctrl Pts',(2.00111428556866,77.7451420947154,22.1006406181192));
#44708=CARTESIAN_POINT('Ctrl Pts',(2.03479950715842,77.786624874732,22.1430856683949));
#44709=CARTESIAN_POINT('Ctrl Pts',(2.08418676443722,77.8526750346387,22.2379141585008));
#44710=CARTESIAN_POINT('Ctrl Pts',(2.10320619628386,77.8816487301738,22.2965714738577));
#44711=CARTESIAN_POINT('Ctrl Pts',(2.12290794061138,77.9202366687201,22.4226781994981));
#44712=CARTESIAN_POINT('Ctrl Pts',(2.12363677900081,77.9298111396176,22.4901325035708));
#44713=CARTESIAN_POINT('Ctrl Pts',(2.11676125496322,77.9298111396176,22.5525394843164));
#44714=CARTESIAN_POINT('',(2.06200638105671,77.9298111396176,23.0495323452143));
#44715=CARTESIAN_POINT('',(2.17151612886973,77.9298111396176,22.0555466234185));
#44716=CARTESIAN_POINT('',(2.31264222801171,78.3249353664633,23.5801708210266));
#44717=CARTESIAN_POINT('Ctrl Pts',(2.06200638105672,77.9298111396176,23.0495323452143));
#44718=CARTESIAN_POINT('Ctrl Pts',(2.05513085701913,77.9298111396176,23.11193932596));
#44719=CARTESIAN_POINT('Ctrl Pts',(2.05592754820022,77.9393273581992,23.1794011055345));
#44720=CARTESIAN_POINT('Ctrl Pts',(2.07509523675738,77.9783737890882,23.305448992993));
#44721=CARTESIAN_POINT('Ctrl Pts',(2.09341990517389,78.0079439461362,23.3640297646265));
#44722=CARTESIAN_POINT('Ctrl Pts',(2.13922834115554,78.0770665607413,23.4584639675621));
#44723=CARTESIAN_POINT('Ctrl Pts',(2.16977139876493,78.1212469206825,23.5005628382322));
#44724=CARTESIAN_POINT('Ctrl Pts',(2.23845975544489,78.2194869113329,23.5594293854225));
#44725=CARTESIAN_POINT('Ctrl Pts',(2.27655500713784,78.2735827563092,23.5761950069173));
#44726=CARTESIAN_POINT('Ctrl Pts',(2.31264222801172,78.3249353664633,23.5801708210266));
#44727=CARTESIAN_POINT('',(3.00123722894601,83.3381380528135,23.6560349539252));
#44728=CARTESIAN_POINT('Origin',(-2.15133476424044,81.5,23.0883639630957));
#44729=CARTESIAN_POINT('',(2.78221773331998,83.3381380528135,25.6440063975169));
#44730=CARTESIAN_POINT('',(3.16550185066553,83.3381380528135,22.1650563712315));
#44731=CARTESIAN_POINT('',(2.09362273238568,78.3249353664633,25.5681422646183));
#44732=CARTESIAN_POINT('Origin',(-2.37035425986648,81.5,25.0763354066873));
#44733=CARTESIAN_POINT('',(1.73347713761766,77.9298111396176,26.0314895106017));
#44734=CARTESIAN_POINT('Ctrl Pts',(2.09362273238568,78.3249353664633,25.5681422646183));
#44735=CARTESIAN_POINT('Ctrl Pts',(2.0575355115118,78.2735827563092,25.5641664505089));
#44736=CARTESIAN_POINT('Ctrl Pts',(2.01670405211226,78.2194869113329,25.5722365303698));
#44737=CARTESIAN_POINT('Ctrl Pts',(1.9368477899923,78.1212469206825,25.6147375670833));
#44738=CARTESIAN_POINT('Ctrl Pts',(1.8978722816583,78.0770665607413,25.6491774136268));
#44739=CARTESIAN_POINT('Ctrl Pts',(1.83260401187277,78.0079439461362,25.7313740343017));
#44740=CARTESIAN_POINT('Ctrl Pts',(1.80196569053251,77.9783737890882,25.7845604380456));
#44741=CARTESIAN_POINT('Ctrl Pts',(1.75581682568182,77.9393273581992,25.9034122469942));
#44742=CARTESIAN_POINT('Ctrl Pts',(1.74035266165525,77.9298111396176,25.9690825298561));
#44743=CARTESIAN_POINT('Ctrl Pts',(1.73347713761766,77.9298111396176,26.0314895106017));
#44744=CARTESIAN_POINT('',(1.67872226371115,77.9298111396176,26.5284823714996));
#44745=CARTESIAN_POINT('',(1.62396738980464,77.9298111396176,27.0254752323975));
#44746=CARTESIAN_POINT('',(1.28413688315078,77.5642538212272,26.9880353051765));
#44747=CARTESIAN_POINT('Ctrl Pts',(1.67872226371115,77.9298111396176,26.5284823714996));
#44748=CARTESIAN_POINT('Ctrl Pts',(1.67184673967356,77.9298111396176,26.5908893522453));
#44749=CARTESIAN_POINT('Ctrl Pts',(1.65645042843866,77.9202366687201,26.656567110609));
#44750=CARTESIAN_POINT('Ctrl Pts',(1.6097675078176,77.8816487301738,26.7753600813757));
#44751=CARTESIAN_POINT('Ctrl Pts',(1.57843442304722,77.8526750346387,26.8284699413964));
#44752=CARTESIAN_POINT('Ctrl Pts',(1.50958733196454,77.786624874732,26.9102722749007));
#44753=CARTESIAN_POINT('Ctrl Pts',(1.46746965965018,77.7451420947154,26.9443659418387));
#44754=CARTESIAN_POINT('Ctrl Pts',(1.37713279980561,77.6558998044384,26.9857123064191));
#44755=CARTESIAN_POINT('Ctrl Pts',(1.32886987540445,77.6081839481971,26.9929636442795));
#44756=CARTESIAN_POINT('Ctrl Pts',(1.28413688315077,77.5642538212272,26.9880353051765));
#44757=CARTESIAN_POINT('Origin',(-2.534618881586,81.5,26.567313989381));
#44758=CARTESIAN_POINT('Origin',(-12.171476686886,81.5,114.038057487035));
#44759=CARTESIAN_POINT('',(-17.0908494176979,81.5,108.465825265084));
#44760=CARTESIAN_POINT('',(-17.6383981567629,81.5,113.435753874063));
#44761=CARTESIAN_POINT('',(-17.6383981567629,81.5,113.435753874063));
#44762=CARTESIAN_POINT('',(-7.80517218308414,77.5642538212272,109.488850193851));
#44763=CARTESIAN_POINT('Origin',(-11.6239279478209,81.5,109.068128878056));
#44764=CARTESIAN_POINT('',(-7.52009655033678,77.9298111396176,110.02328298197));
#44765=CARTESIAN_POINT('Ctrl Pts',(-7.80517218308414,77.5642538212272,109.488850193851));
#44766=CARTESIAN_POINT('Ctrl Pts',(-7.76043919083047,77.6081839481971,109.493778532954));
#44767=CARTESIAN_POINT('Ctrl Pts',(-7.7149124741359,77.6558998044383,109.51136289645));
#44768=CARTESIAN_POINT('Ctrl Pts',(-7.63574351973134,77.7451420947154,109.571384115773));
#44769=CARTESIAN_POINT('Ctrl Pts',(-7.60205829814157,77.786624874732,109.613829166049));
#44770=CARTESIAN_POINT('Ctrl Pts',(-7.55267104086277,77.8526750346387,109.708657656155));
#44771=CARTESIAN_POINT('Ctrl Pts',(-7.53365160901614,77.8816487301738,109.767314971512));
#44772=CARTESIAN_POINT('Ctrl Pts',(-7.51394986468862,77.9202366687201,109.893421697152));
#44773=CARTESIAN_POINT('Ctrl Pts',(-7.5132210262992,77.9298111396176,109.960876001225));
#44774=CARTESIAN_POINT('Ctrl Pts',(-7.52009655033678,77.9298111396176,110.02328298197));
#44775=CARTESIAN_POINT('',(-7.57485142424329,77.9298111396176,110.520275842868));
#44776=CARTESIAN_POINT('',(-7.46534167643027,77.9298111396176,109.526290121073));
#44777=CARTESIAN_POINT('',(-7.32421557728829,78.3249353664633,111.050914318681));
#44778=CARTESIAN_POINT('Ctrl Pts',(-7.57485142424328,77.9298111396176,110.520275842868));
#44779=CARTESIAN_POINT('Ctrl Pts',(-7.58172694828087,77.9298111396176,110.582682823614));
#44780=CARTESIAN_POINT('Ctrl Pts',(-7.58093025709977,77.9393273581992,110.650144603188));
#44781=CARTESIAN_POINT('Ctrl Pts',(-7.56176256854262,77.9783737890883,110.776192490647));
#44782=CARTESIAN_POINT('Ctrl Pts',(-7.54343790012612,78.0079439461362,110.834773262281));
#44783=CARTESIAN_POINT('Ctrl Pts',(-7.49762946414447,78.0770665607413,110.929207465216));
#44784=CARTESIAN_POINT('Ctrl Pts',(-7.46708640653507,78.1212469206825,110.971306335886));
#44785=CARTESIAN_POINT('Ctrl Pts',(-7.39839804985511,78.2194869113329,111.030172883077));
#44786=CARTESIAN_POINT('Ctrl Pts',(-7.36030279816216,78.2735827563092,111.046938504571));
#44787=CARTESIAN_POINT('Ctrl Pts',(-7.32421557728828,78.3249353664633,111.050914318681));
#44788=CARTESIAN_POINT('',(-6.63562057635399,83.3381380528135,111.126778451579));
#44789=CARTESIAN_POINT('Origin',(-11.7881925695404,81.5,110.55910746075));
#44790=CARTESIAN_POINT('',(-6.85464007198003,83.3381380528135,113.114749895171));
#44791=CARTESIAN_POINT('',(-6.47135595463447,83.3381380528135,109.635799868886));
#44792=CARTESIAN_POINT('',(-7.54323507291432,78.3249353664633,113.038885762272));
#44793=CARTESIAN_POINT('Origin',(-12.0072120651665,81.5,112.547078904341));
#44794=CARTESIAN_POINT('',(-7.90338066768234,77.9298111396176,113.502233008256));
#44795=CARTESIAN_POINT('Ctrl Pts',(-7.54323507291431,78.3249353664633,113.038885762272));
#44796=CARTESIAN_POINT('Ctrl Pts',(-7.57932229378819,78.2735827563092,113.034909948163));
#44797=CARTESIAN_POINT('Ctrl Pts',(-7.62015375318775,78.2194869113329,113.042980028024));
#44798=CARTESIAN_POINT('Ctrl Pts',(-7.7000100153077,78.1212469206825,113.085481064737));
#44799=CARTESIAN_POINT('Ctrl Pts',(-7.7389855236417,78.0770665607413,113.119920911281));
#44800=CARTESIAN_POINT('Ctrl Pts',(-7.80425379342723,78.0079439461362,113.202117531956));
#44801=CARTESIAN_POINT('Ctrl Pts',(-7.83489211476748,77.9783737890882,113.2553039357));
#44802=CARTESIAN_POINT('Ctrl Pts',(-7.88104097961818,77.9393273581992,113.374155744648));
#44803=CARTESIAN_POINT('Ctrl Pts',(-7.89650514364476,77.9298111396176,113.43982602751));
#44804=CARTESIAN_POINT('Ctrl Pts',(-7.90338066768234,77.9298111396176,113.502233008256));
#44805=CARTESIAN_POINT('',(-7.95813554158885,77.9298111396176,113.999225869154));
#44806=CARTESIAN_POINT('',(-8.01289041549536,77.9298111396176,114.496218730052));
#44807=CARTESIAN_POINT('',(-8.35272092214922,77.5642538212272,114.45877880283));
#44808=CARTESIAN_POINT('Ctrl Pts',(-7.95813554158885,77.9298111396176,113.999225869154));
#44809=CARTESIAN_POINT('Ctrl Pts',(-7.96501106562644,77.9298111396176,114.061632849899));
#44810=CARTESIAN_POINT('Ctrl Pts',(-7.98040737686134,77.9202366687201,114.127310608263));
#44811=CARTESIAN_POINT('Ctrl Pts',(-8.0270902974824,77.8816487301738,114.24610357903));
#44812=CARTESIAN_POINT('Ctrl Pts',(-8.0584233822528,77.8526750346387,114.29921343905));
#44813=CARTESIAN_POINT('Ctrl Pts',(-8.12727047333548,77.786624874732,114.381015772555));
#44814=CARTESIAN_POINT('Ctrl Pts',(-8.16938814564984,77.7451420947154,114.415109439493));
#44815=CARTESIAN_POINT('Ctrl Pts',(-8.25972500549441,77.6558998044383,114.456455804073));
#44816=CARTESIAN_POINT('Ctrl Pts',(-8.30798792989556,77.6081839481971,114.463707141934));
#44817=CARTESIAN_POINT('Ctrl Pts',(-8.35272092214923,77.5642538212272,114.45877880283));
#44818=CARTESIAN_POINT('Origin',(-12.171476686886,81.5,114.038057487035));
#44819=CARTESIAN_POINT('Origin',(-14.7997106497322,77.000000018974,137.893714808445));
#44820=CARTESIAN_POINT('',(-17.0067015889499,77.000000018974,139.662666756411));
#44821=CARTESIAN_POINT('Origin',(-15.0187301453583,77.000000018974,139.881686252037));
#44822=CARTESIAN_POINT('',(-16.7876820933239,77.000000018974,137.674695312819));
#44823=CARTESIAN_POINT('',(-16.7876820933239,77.000000018974,137.674695312819));
#44824=CARTESIAN_POINT('Origin',(-14.7997106497322,77.000000018974,137.893714808445));
#44825=CARTESIAN_POINT('Origin',(-11.2953987197157,81.500000018974,106.086171710979));
#44826=CARTESIAN_POINT('',(-13.7803630242052,81.500000018974,105.812397341447));
#44827=CARTESIAN_POINT('Origin',(-11.2953987197157,81.500000018974,106.086171710979));
#44828=CARTESIAN_POINT('',(-15.0944799979614,81.500000018974,117.740226002996));
#44829=CARTESIAN_POINT('',(-13.7803630242052,81.500000018974,105.812397341447));
#44830=CARTESIAN_POINT('Origin',(-12.6095156934719,81.500000018974,118.014000372529));
#44831=CARTESIAN_POINT('Origin',(-12.5547608195654,81.500000018974,117.517007511631));
#44832=CARTESIAN_POINT('',(-9.55592370657306,81.500000018974,106.277813769652));
#44833=CARTESIAN_POINT('Origin',(-11.2953987197157,81.500000018974,106.086171710979));
#44834=CARTESIAN_POINT('',(-10.8152858064227,81.500000018974,117.708649570304));
#44835=CARTESIAN_POINT('',(-10.8152858064227,81.500000018974,117.708649570304));
#44836=CARTESIAN_POINT('Origin',(-12.5547608195654,81.500000018974,117.517007511631));
#44837=CARTESIAN_POINT('Origin',(-7.01890469369955,83.3381380528135,114.605728477865));
#44838=CARTESIAN_POINT('',(-7.13261343725189,84.204163456598,111.072023577673));
#44839=CARTESIAN_POINT('',(-7.57245184784244,83.0039311341202,111.023565544156));
#44840=CARTESIAN_POINT('Origin',(-6.63562057635399,83.3381380528135,111.126778451579));
#44841=CARTESIAN_POINT('',(-7.79147134346847,83.0039311341202,113.011536987747));
#44842=CARTESIAN_POINT('',(-7.955735965188,83.0039311341202,114.502515570441));
#44843=CARTESIAN_POINT('',(-7.35163293287793,84.204163456598,113.059995021264));
#44844=CARTESIAN_POINT('Origin',(-6.85464007198003,83.3381380528135,113.114749895171));
#44845=CARTESIAN_POINT('',(-7.51589755459745,84.204163456598,114.550973603958));
#44846=CARTESIAN_POINT('Origin',(-7.01890469369955,79.6618619471865,114.605728477865));
#44847=CARTESIAN_POINT('',(-7.37353488244054,78.795836543402,113.258792165624));
#44848=CARTESIAN_POINT('Origin',(-6.87654202154263,79.6618619471865,113.31354703953));
#44849=CARTESIAN_POINT('',(-7.51589755459745,78.795836543402,114.550973603958));
#44850=CARTESIAN_POINT('',(-7.51589755459745,78.795836543402,114.550973603958));
#44851=CARTESIAN_POINT('Origin',(-7.01890469369955,79.6618619471865,114.605728477865));
#44852=CARTESIAN_POINT('Origin',(-7.01890469369955,79.6618619471865,114.605728477865));
#44853=CARTESIAN_POINT('',(-6.96834881553237,78.795836543402,109.581044994979));
#44854=CARTESIAN_POINT('Origin',(-6.47135595463447,79.6618619471865,109.635799868886));
#44855=CARTESIAN_POINT('',(-7.1107114876893,78.795836543402,110.873226433314));
#44856=CARTESIAN_POINT('',(-7.51589755459745,78.795836543402,114.550973603958));
#44857=CARTESIAN_POINT('Origin',(-6.61371862679139,79.6618619471865,110.92798130722));
#44858=CARTESIAN_POINT('Origin',(-12.171476686886,81.5,114.038057487035));
#44859=CARTESIAN_POINT('',(-7.01890469369955,79.6618619471865,114.605728477865));
#44860=CARTESIAN_POINT('Origin',(-12.171476686886,81.5,114.038057487035));
#44861=CARTESIAN_POINT('',(-6.87654202154265,79.6618619471864,113.31354703953));
#44862=CARTESIAN_POINT('',(-6.47135595463447,79.6618619471865,109.635799868886));
#44863=CARTESIAN_POINT('',(-12.0291140147291,87.,112.7458760487));
#44864=CARTESIAN_POINT('Origin',(-12.0291140147291,81.5,112.7458760487));
#44865=CARTESIAN_POINT('',(-11.7662906199778,87.,110.360310316391));
#44866=CARTESIAN_POINT('',(-12.0291140147291,87.,112.7458760487));
#44867=CARTESIAN_POINT('',(-6.61371862679139,79.6618619471865,110.92798130722));
#44868=CARTESIAN_POINT('Origin',(-11.7662906199778,81.5,110.360310316391));
#44869=CARTESIAN_POINT('',(-6.47135595463447,79.6618619471865,109.635799868886));
#44870=CARTESIAN_POINT('',(-6.47135595463447,79.6618619471865,109.635799868886));
#44871=CARTESIAN_POINT('Origin',(-11.6239279478209,81.5,109.068128878056));
#44872=CARTESIAN_POINT('Origin',(2.61795311160045,79.6618619471865,27.1349849802106));
#44873=CARTESIAN_POINT('',(2.26332292285946,78.795836543402,25.7880486679695));
#44874=CARTESIAN_POINT('Origin',(2.76031578375737,79.6618619471865,25.842803541876));
#44875=CARTESIAN_POINT('',(2.12096025070255,78.795836543402,27.0802301063041));
#44876=CARTESIAN_POINT('',(2.12096025070255,78.795836543402,27.0802301063041));
#44877=CARTESIAN_POINT('Origin',(2.61795311160045,79.6618619471865,27.1349849802106));
#44878=CARTESIAN_POINT('Origin',(2.61795311160045,79.6618619471865,27.1349849802106));
#44879=CARTESIAN_POINT('',(2.66850898976763,78.795836543402,22.110301497325));
#44880=CARTESIAN_POINT('Origin',(3.16550185066553,79.6618619471865,22.1650563712315));
#44881=CARTESIAN_POINT('',(2.5261463176107,78.795836543402,23.4024829356596));
#44882=CARTESIAN_POINT('',(2.12096025070255,78.795836543402,27.0802301063041));
#44883=CARTESIAN_POINT('Origin',(3.02313917850861,79.6618619471865,23.4572378095661));
#44884=CARTESIAN_POINT('Origin',(-2.534618881586,81.5,26.567313989381));
#44885=CARTESIAN_POINT('',(2.61795311160045,79.6618619471865,27.1349849802106));
#44886=CARTESIAN_POINT('Origin',(-2.534618881586,81.5,26.567313989381));
#44887=CARTESIAN_POINT('',(2.76031578375735,79.6618619471864,25.842803541876));
#44888=CARTESIAN_POINT('',(3.16550185066553,79.6618619471865,22.1650563712315));
#44889=CARTESIAN_POINT('',(-2.39225620942908,87.,25.2751325510465));
#44890=CARTESIAN_POINT('Origin',(-2.39225620942908,81.5,25.2751325510465));
#44891=CARTESIAN_POINT('',(-2.12943281467784,87.,22.8895668187365));
#44892=CARTESIAN_POINT('',(-2.39225620942908,87.,25.2751325510465));
#44893=CARTESIAN_POINT('',(3.02313917850861,79.6618619471865,23.4572378095661));
#44894=CARTESIAN_POINT('Origin',(-2.12943281467784,81.5,22.8895668187365));
#44895=CARTESIAN_POINT('',(3.16550185066553,79.6618619471865,22.1650563712315));
#44896=CARTESIAN_POINT('',(3.16550185066553,79.6618619471865,22.1650563712315));
#44897=CARTESIAN_POINT('Origin',(-1.98707014252092,81.5,21.597385380402));
#44898=CARTESIAN_POINT('Origin',(2.61795311160045,83.3381380528135,27.1349849802106));
#44899=CARTESIAN_POINT('',(2.50424436804811,84.204163456598,23.6012800800187));
#44900=CARTESIAN_POINT('Origin',(3.00123722894601,83.3381380528135,23.6560349539252));
#44901=CARTESIAN_POINT('',(2.28522487242207,84.204163456598,25.5892515236103));
#44902=CARTESIAN_POINT('Origin',(2.78221773331998,83.3381380528135,25.6440063975169));
#44903=CARTESIAN_POINT('',(2.12096025070255,84.204163456598,27.0802301063041));
#44904=CARTESIAN_POINT('Origin',(-12.6095156787167,81.500000021449,118.014000374155));
#44905=CARTESIAN_POINT('',(1.82040912887033,81.500000021449,18.9987123119195));
#44906=CARTESIAN_POINT('Origin',(-1.658540897415,81.500000021449,18.615428194574));
#44907=CARTESIAN_POINT('',(-9.13056565243138,81.500000021449,118.3972844915));
#44908=CARTESIAN_POINT('',(-9.13056565243138,81.500000021449,118.3972844915));
#44909=CARTESIAN_POINT('Origin',(-12.6095156787167,81.500000021449,118.014000374155));
#44910=CARTESIAN_POINT('Origin',(-12.6095156787167,81.500000021449,118.014000374155));
#44911=CARTESIAN_POINT('Origin',(-12.0072120651665,81.5,112.547078904341));
#44912=CARTESIAN_POINT('Origin',(-11.7881925695404,81.5,110.55910746075));
#44913=CARTESIAN_POINT('',(-11.7662906199778,86.0000000007944,110.36031031639));
#44914=CARTESIAN_POINT('Origin',(-11.7662906199778,81.5,110.360310316391));
#44915=CARTESIAN_POINT('',(-12.0291140147291,86.0000000007944,112.7458760487));
#44916=CARTESIAN_POINT('',(-11.7662906199778,86.,110.360310316391));
#44917=CARTESIAN_POINT('Origin',(-12.0291140147291,81.5,112.7458760487));
#44918=CARTESIAN_POINT('Origin',(-1.658540897415,81.500000021449,18.615428194574));
#44919=CARTESIAN_POINT('Origin',(0.918613714880988,78.570620200579,26.5704957561906));
#44920=CARTESIAN_POINT('',(0.987057307264123,78.570620200579,25.9492546800682));
#44921=CARTESIAN_POINT('',(0.932302433357615,78.570620200579,26.4462475409661));
#44922=CARTESIAN_POINT('Origin',(1.38403014308631,78.570620200579,22.3460564385584));
#44923=CARTESIAN_POINT('',(1.36065466016491,78.5789363869598,22.4692374401316));
#44924=CARTESIAN_POINT('',(1.31558655070317,78.570620200579,22.9672975146808));
#44925=CARTESIAN_POINT('Origin',(4.9436803483069,84.8504809471617,25.3791144897641));
#44926=CARTESIAN_POINT('',(4.51618082872696,85.5,25.8350411952321));
#44927=CARTESIAN_POINT('',(5.00134414567056,85.75,25.3854674461182));
#44928=CARTESIAN_POINT('Origin',(4.57093570263347,85.5,25.3380483343342));
#44929=CARTESIAN_POINT('',(5.01317368962486,84.6339745962156,25.8897960691386));
#44930=CARTESIAN_POINT('',(5.01317368962486,84.6339745962156,25.8897960691386));
#44931=CARTESIAN_POINT('',(5.49833700656846,84.8839745962156,25.4402223200247));
#44932=CARTESIAN_POINT('Origin',(5.06792856353137,84.6339745962156,25.3928032082407));
#44933=CARTESIAN_POINT('',(5.37408879134399,85.1004809471617,25.4265336015481));
#44934=CARTESIAN_POINT('Origin',(5.44358213266196,84.8839745962156,25.9372151809226));
#44935=CARTESIAN_POINT('',(0.812803082748461,79.4245321397111,25.4270313474792));
#44936=CARTESIAN_POINT('',(5.44358213266196,84.8839745962156,25.9372151809226));
#44937=CARTESIAN_POINT('',(2.28522487242207,84.204163456598,25.5892515236103));
#44938=CARTESIAN_POINT('Origin',(2.12096025070255,84.204163456598,27.0802301063041));
#44939=CARTESIAN_POINT('',(5.11085389348358,85.75,24.3914817243224));
#44940=CARTESIAN_POINT('',(4.78232465004453,85.75,27.3734388897098));
#44941=CARTESIAN_POINT('',(4.73520032435299,85.5,23.8470697516405));
#44942=CARTESIAN_POINT('Origin',(4.68044545044649,85.5,24.3440626125384));
#44943=CARTESIAN_POINT('',(2.50424436804811,84.204163456598,23.6012800800187));
#44944=CARTESIAN_POINT('Origin',(0.758048208841953,79.4245321397111,25.9240242083771));
#44945=CARTESIAN_POINT('Origin',(-6.46000589060205,81.5,21.1045915152434));
#44946=CARTESIAN_POINT('',(1.84890551511204,77.5494703669995,22.0200038523508));
#44947=CARTESIAN_POINT('',(5.39645780697042,78.3660254037844,22.4108460428533));
#44948=CARTESIAN_POINT('',(5.82686625000751,78.1160254037844,22.4582651546373));
#44949=CARTESIAN_POINT('',(4.89946494607252,77.5,22.3560911689468));
#44950=CARTESIAN_POINT('',(4.89946494607252,77.5,22.3560911689468));
#44951=CARTESIAN_POINT('',(5.32987338910961,77.25,22.4035102807308));
#44952=CARTESIAN_POINT('Origin',(5.17743831134439,84.6339745962156,24.3988174864449));
#44953=CARTESIAN_POINT('',(5.60784675438148,84.8839745962156,24.4462365982289));
#44954=CARTESIAN_POINT('',(5.11085389348358,85.75,24.3914817243224));
#44955=CARTESIAN_POINT('',(5.2321931852509,84.6339745962156,23.901824625547));
#44956=CARTESIAN_POINT('Origin',(5.17743831134439,84.6339745962156,24.3988174864449));
#44957=CARTESIAN_POINT('',(5.2321931852509,84.6339745962156,23.901824625547));
#44958=CARTESIAN_POINT('Origin',(1.63819716446086,78.9509609731971,23.0028402857485));
#44959=CARTESIAN_POINT('',(1.03182257837449,79.4245321397111,23.4390599038876));
#44960=CARTESIAN_POINT('Origin',(-5.96583445235644,83.8354360064825,25.6862635551102));
#44961=CARTESIAN_POINT('',(-6.02058932626295,83.8354360064825,26.1832564160081));
#44962=CARTESIAN_POINT('Origin',(-8.00154035146294,81.5,25.9650103764094));
#44963=CARTESIAN_POINT('',(4.35191620700744,77.5,27.3260197779258));
#44964=CARTESIAN_POINT('',(4.78232465004453,77.25,27.3734388897098));
#44965=CARTESIAN_POINT('',(4.84890906790534,78.3660254037844,27.3807746518323));
#44966=CARTESIAN_POINT('',(4.84890906790534,78.3660254037844,27.3807746518323));
#44967=CARTESIAN_POINT('',(5.27931751094243,78.1160254037844,27.4281937636163));
#44968=CARTESIAN_POINT('Origin',(3.16550185066553,83.3381380528135,22.1650563712315));
#44969=CARTESIAN_POINT('',(5.66260162828799,84.8839745962156,23.949243737331));
#44970=CARTESIAN_POINT('',(5.82686625000751,84.8839745962156,22.4582651546373));
#44971=CARTESIAN_POINT('Origin',(5.66260162828799,84.8839745962156,23.949243737331));
#44972=CARTESIAN_POINT('Origin',(1.04773081085198,78.1902794279609,22.4347618827151));
#44973=CARTESIAN_POINT('Origin',(5.29195648048422,85.1004809471617,26.172022892895));
#44974=CARTESIAN_POINT('Origin',(-2.19513866336565,86.75,23.485958251814));
#44975=CARTESIAN_POINT('',(-2.39225620942908,86.,25.2751325510465));
#44976=CARTESIAN_POINT('',(-2.12943281467784,87.,22.8895668187365));
#44977=CARTESIAN_POINT('Origin',(4.90366394181185,78.3660254037844,26.8837817909344));
#44978=CARTESIAN_POINT('',(4.83707952395104,77.25,26.8764460288119));
#44979=CARTESIAN_POINT('Origin',(4.40667108091395,77.5,26.8290269170279));
#44980=CARTESIAN_POINT('',(5.33407238484894,78.1160254037844,26.9312009027185));
#44981=CARTESIAN_POINT('',(5.20982416962446,77.8995190528383,26.9175121842418));
#44982=CARTESIAN_POINT('Origin',(4.90366394181185,78.3660254037844,26.8837817909344));
#44983=CARTESIAN_POINT('Origin',(5.29195648048422,77.8995190528383,26.172022892895));
#44984=CARTESIAN_POINT('',(5.2751185152031,77.25,22.9005031416287));
#44985=CARTESIAN_POINT('',(4.78232465004453,77.25,27.3734388897098));
#44986=CARTESIAN_POINT('',(5.772111376101,78.1160254037844,22.9552580155352));
#44987=CARTESIAN_POINT('',(5.64786316087653,77.8995190528383,22.9415692970586));
#44988=CARTESIAN_POINT('',(5.82686625000751,78.1160254037844,22.4582651546373));
#44989=CARTESIAN_POINT('Origin',(5.82686625000751,78.1160254037844,22.4582651546373));
#44990=CARTESIAN_POINT('Origin',(5.34170293306391,78.3660254037844,22.9078389037512));
#44991=CARTESIAN_POINT('',(4.3538213781796,78.8889436754855,23.603842201269));
#44992=CARTESIAN_POINT('',(3.02313917850861,79.6618619471865,23.4572378095661));
#44993=CARTESIAN_POINT('',(4.09099798342836,78.8889436754855,25.9894079335789));
#44994=CARTESIAN_POINT('',(4.09099798342836,78.8889436754855,25.9894079335789));
#44995=CARTESIAN_POINT('',(2.76031578375737,79.6618619471865,25.842803541876));
#44996=CARTESIAN_POINT('Origin',(4.16386731426731,78.6724373245393,24.1865449158698));
#44997=CARTESIAN_POINT('',(3.85682851728169,78.022918271701,23.5490873273625));
#44998=CARTESIAN_POINT('',(4.3538213781796,78.8889436754855,23.603842201269));
#44999=CARTESIAN_POINT('',(3.59400512253045,78.022918271701,25.9346530596724));
#45000=CARTESIAN_POINT('',(3.85682851728169,78.022918271701,23.5490873273625));
#45001=CARTESIAN_POINT('',(3.59400512253045,78.022918271701,25.9346530596724));
#45002=CARTESIAN_POINT('Origin',(-2.12943281467784,87.,22.8895668187365));
#45003=CARTESIAN_POINT('',(2.52614631761071,78.795836543402,23.4024829356596));
#45004=CARTESIAN_POINT('Origin',(4.78232465004453,77.25,27.3734388897098));
#45005=CARTESIAN_POINT('Origin',(4.84471007216601,77.5,22.8530840298447));
#45006=CARTESIAN_POINT('',(2.26332292285947,78.795836543402,25.7880486679695));
#45007=CARTESIAN_POINT('Origin',(-2.39225620942908,86.,25.2751325510465));
#45008=CARTESIAN_POINT('Origin',(4.84471007216601,77.5,22.8530840298447));
#45009=CARTESIAN_POINT('Origin',(-11.8319964686657,86.75,110.956701749468));
#45010=CARTESIAN_POINT('',(-12.0291140147291,86.,112.7458760487));
#45011=CARTESIAN_POINT('',(-11.7662906199778,87.,110.360310316391));
#45012=CARTESIAN_POINT('Origin',(-4.73319386348815,78.3660254037844,114.354525288588));
#45013=CARTESIAN_POINT('',(-4.79977828134896,77.25,114.347189526466));
#45014=CARTESIAN_POINT('',(-5.28494159829256,77.5,114.79676327558));
#45015=CARTESIAN_POINT('Origin',(-5.23018672438606,77.5,114.299770414682));
#45016=CARTESIAN_POINT('',(-4.30278542045106,78.1160254037844,114.401944400372));
#45017=CARTESIAN_POINT('',(-4.42703363567554,77.8995190528383,114.388255681896));
#45018=CARTESIAN_POINT('',(-4.78794873739466,78.3660254037844,114.851518149486));
#45019=CARTESIAN_POINT('Origin',(-4.73319386348815,78.3660254037844,114.354525288588));
#45020=CARTESIAN_POINT('',(-4.78794873739466,78.3660254037844,114.851518149486));
#45021=CARTESIAN_POINT('Origin',(-4.34490132481578,77.8995190528383,113.642766390549));
#45022=CARTESIAN_POINT('',(-4.3617392900969,77.25,110.371246639283));
#45023=CARTESIAN_POINT('',(-4.85453315525547,77.25,114.844182387364));
#45024=CARTESIAN_POINT('',(-3.864746429199,78.1160254037844,110.426001513189));
#45025=CARTESIAN_POINT('',(-3.98899464442347,77.8995190528383,110.412312794713));
#45026=CARTESIAN_POINT('',(-3.80999155529249,78.1160254037844,109.929008652291));
#45027=CARTESIAN_POINT('Origin',(-3.80999155529249,78.1160254037844,109.929008652291));
#45028=CARTESIAN_POINT('',(-4.24039999832958,78.3660254037844,109.881589540507));
#45029=CARTESIAN_POINT('Origin',(-4.29515487223609,78.3660254037844,110.378582401405));
#45030=CARTESIAN_POINT('',(-3.80999155529249,78.1160254037844,109.929008652291));
#45031=CARTESIAN_POINT('',(-5.28303642712041,78.8889436754855,111.074585698923));
#45032=CARTESIAN_POINT('',(-6.61371862679139,79.6618619471865,110.92798130722));
#45033=CARTESIAN_POINT('',(-5.54585982187164,78.8889436754855,113.460151431233));
#45034=CARTESIAN_POINT('',(-5.54585982187164,78.8889436754855,113.460151431233));
#45035=CARTESIAN_POINT('',(-6.87654202154263,79.6618619471865,113.31354703953));
#45036=CARTESIAN_POINT('',(-4.35754029435757,78.1160254037844,114.89893726127));
#45037=CARTESIAN_POINT('Origin',(-5.47299049103269,78.6724373245393,111.657288413524));
#45038=CARTESIAN_POINT('',(-5.78002928801831,78.022918271701,111.019830825016));
#45039=CARTESIAN_POINT('',(-5.28303642712041,78.8889436754855,111.074585698923));
#45040=CARTESIAN_POINT('',(-6.04285268276955,78.022918271701,113.405396557326));
#45041=CARTESIAN_POINT('',(-5.78002928801831,78.022918271701,111.019830825016));
#45042=CARTESIAN_POINT('',(-6.04285268276955,78.022918271701,113.405396557326));
#45043=CARTESIAN_POINT('Origin',(-11.7662906199778,87.,110.360310316391));
#45044=CARTESIAN_POINT('',(-7.11071148768929,78.795836543402,110.873226433314));
#45045=CARTESIAN_POINT('Origin',(-4.85453315525547,77.25,114.844182387364));
#45046=CARTESIAN_POINT('',(-4.73739285922748,77.5,109.826834666601));
#45047=CARTESIAN_POINT('',(-4.30698441619039,77.25,109.874253778385));
#45048=CARTESIAN_POINT('Origin',(-4.79214773313399,77.5,110.323827527499));
#45049=CARTESIAN_POINT('',(-4.85453315525547,77.25,114.844182387364));
#45050=CARTESIAN_POINT('',(-7.37353488244053,78.795836543402,113.258792165624));
#45051=CARTESIAN_POINT('Origin',(-4.30698441619039,77.25,109.874253778385));
#45052=CARTESIAN_POINT('',(-4.73739285922748,77.5,109.826834666601));
#45053=CARTESIAN_POINT('',(-7.78795229018796,77.5494703669995,109.490747350005));
#45054=CARTESIAN_POINT('Origin',(-4.35754029435757,78.1160254037844,114.89893726127));
#45055=CARTESIAN_POINT('',(-15.657447131563,83.8354360064825,113.653999913662));
#45056=CARTESIAN_POINT('Origin',(-12.0291140147291,86.,112.7458760487));
#45057=CARTESIAN_POINT('Origin',(-4.79214773313399,77.5,110.323827527499));
#45058=CARTESIAN_POINT('Origin',(-8.71824409041901,78.570620200579,114.041239253845));
#45059=CARTESIAN_POINT('',(-8.64980049803588,78.570620200579,113.419998177722));
#45060=CARTESIAN_POINT('',(-8.70455537194238,78.570620200579,113.91699103862));
#45061=CARTESIAN_POINT('Origin',(-8.25282766221369,78.570620200579,109.816799936212));
#45062=CARTESIAN_POINT('',(-8.27620314513509,78.5789363869598,109.939980937786));
#45063=CARTESIAN_POINT('',(-8.32127125459683,78.570620200579,110.438041012335));
#45064=CARTESIAN_POINT('Origin',(-4.6931774569931,84.8504809471617,112.849857987418));
#45065=CARTESIAN_POINT('',(-5.12067697657304,85.5,113.305784692886));
#45066=CARTESIAN_POINT('',(-4.63551365962944,85.75,112.856210943772));
#45067=CARTESIAN_POINT('Origin',(-5.06592210266653,85.5,112.808791831988));
#45068=CARTESIAN_POINT('',(-4.62368411567514,84.6339745962156,113.360539566793));
#45069=CARTESIAN_POINT('',(-4.62368411567514,84.6339745962156,113.360539566793));
#45070=CARTESIAN_POINT('',(-4.13852079873154,84.8839745962156,112.910965817679));
#45071=CARTESIAN_POINT('Origin',(-4.56892924176863,84.6339745962156,112.863546705895));
#45072=CARTESIAN_POINT('',(-4.26276901395601,85.1004809471617,112.897277099202));
#45073=CARTESIAN_POINT('Origin',(-4.19327567263805,84.8839745962156,113.407958678577));
#45074=CARTESIAN_POINT('',(-8.82405472255154,79.4245321397111,112.897774845133));
#45075=CARTESIAN_POINT('',(-4.19327567263805,84.8839745962156,113.407958678577));
#45076=CARTESIAN_POINT('',(-7.35163293287793,84.204163456598,113.059995021264));
#45077=CARTESIAN_POINT('Origin',(-7.51589755459745,84.204163456598,114.550973603958));
#45078=CARTESIAN_POINT('',(-4.52600391181642,85.75,111.862225221976));
#45079=CARTESIAN_POINT('',(-4.85453315525547,85.75,114.844182387364));
#45080=CARTESIAN_POINT('',(-4.90165748094701,85.5,111.317813249294));
#45081=CARTESIAN_POINT('Origin',(-4.95641235485351,85.5,111.814806110192));
#45082=CARTESIAN_POINT('',(-7.13261343725189,84.204163456598,111.072023577673));
#45083=CARTESIAN_POINT('Origin',(-8.87880959645805,79.4245321397111,113.394767706031));
#45084=CARTESIAN_POINT('Origin',(-4.45941949395561,84.6339745962156,111.869560984099));
#45085=CARTESIAN_POINT('',(-4.02901105091852,84.8839745962156,111.916980095883));
#45086=CARTESIAN_POINT('',(-4.52600391181642,85.75,111.862225221976));
#45087=CARTESIAN_POINT('',(-4.4046646200491,84.6339745962156,111.372568123201));
#45088=CARTESIAN_POINT('Origin',(-4.45941949395561,84.6339745962156,111.869560984099));
#45089=CARTESIAN_POINT('',(-4.4046646200491,84.6339745962156,111.372568123201));
#45090=CARTESIAN_POINT('Origin',(-7.99866064083914,78.9509609731971,110.473583783403));
#45091=CARTESIAN_POINT('',(-8.60503522692551,79.4245321397111,110.909803401542));
#45092=CARTESIAN_POINT('Origin',(-15.6026922576564,83.8354360064825,113.157007052764));
#45093=CARTESIAN_POINT('Origin',(-6.47135595463447,83.3381380528135,109.635799868886));
#45094=CARTESIAN_POINT('',(-3.97425617701201,84.8839745962156,111.419987234985));
#45095=CARTESIAN_POINT('',(-3.80999155529249,84.8839745962156,109.929008652291));
#45096=CARTESIAN_POINT('Origin',(-3.97425617701201,84.8839745962156,111.419987234985));
#45097=CARTESIAN_POINT('Origin',(-8.58912699444802,78.1902794279609,109.905505380369));
#45098=CARTESIAN_POINT('Origin',(-4.34490132481578,85.1004809471617,113.642766390549));
#45099=CARTESIAN_POINT('Origin',(-12.5547608195654,81.500000018974,117.517007511631));
#45100=CARTESIAN_POINT('Origin',(-11.2953987197157,81.500000018974,106.086171710979));
#45101=CARTESIAN_POINT('Origin',(-12.6095156934719,81.500000018974,118.014000372529));
#45102=CARTESIAN_POINT('Origin',(-14.7997106497322,77.000000018974,137.893714808445));
#45103=CARTESIAN_POINT('Origin',(-4.40913348865652,75.500000018974,118.917455791986));
#45104=CARTESIAN_POINT('',(-4.9566822277216,75.500000018974,123.887384400965));
#45105=CARTESIAN_POINT('',(-21.3574466373524,75.500000018974,122.080473562051));
#45106=CARTESIAN_POINT('',(-4.9566822277216,75.500000018974,123.887384400965));
#45107=CARTESIAN_POINT('',(-20.8098978982873,75.500000018974,117.110544953072));
#45108=CARTESIAN_POINT('',(-20.8098978982873,75.500000018974,117.110544953072));
#45109=CARTESIAN_POINT('',(-4.40913348865652,75.500000018974,118.917455791986));
#45110=CARTESIAN_POINT('',(-4.40913348865652,75.500000018974,118.917455791986));
#45111=CARTESIAN_POINT('',(-4.40913348865652,75.500000018974,118.917455791986));
#45112=CARTESIAN_POINT('Origin',(-20.8098978982873,75.500000018974,117.110544953072));
#45113=CARTESIAN_POINT('',(-21.3574466373524,87.500000018974,122.080473562051));
#45114=CARTESIAN_POINT('',(-21.3574466373524,75.500000018974,122.080473562051));
#45115=CARTESIAN_POINT('',(-20.8098978982873,87.500000018974,117.110544953072));
#45116=CARTESIAN_POINT('',(-20.8098978982873,87.500000018974,117.110544953072));
#45117=CARTESIAN_POINT('',(-20.8098978982873,75.500000018974,117.110544953072));
#45118=CARTESIAN_POINT('Origin',(-6.07285864919602,72.500000018974,140.867273982354));
#45119=CARTESIAN_POINT('',(-4.21119293637475,73.000000018974,123.969516711825));
#45120=CARTESIAN_POINT('',(-4.21119293637475,90.000000018974,123.969516711825));
#45121=CARTESIAN_POINT('',(-4.21119293637475,72.500000018974,123.969516711825));
#45122=CARTESIAN_POINT('',(-6.07285864919602,90.000000018974,140.867273982354));
#45123=CARTESIAN_POINT('',(-6.07285864919602,90.000000018974,140.867273982354));
#45124=CARTESIAN_POINT('',(-6.07285864919602,73.000000018974,140.867273982354));
#45125=CARTESIAN_POINT('',(-6.07285864919602,72.500000018974,140.867273982354));
#45126=CARTESIAN_POINT('',(-6.07285864919602,73.000000018974,140.867273982354));
#45127=CARTESIAN_POINT('Origin',(-6.56985151009392,73.000000018974,140.812519108447));
#45128=CARTESIAN_POINT('',(-6.56985151009392,72.500000018974,140.812519108447));
#45129=CARTESIAN_POINT('Origin',(-6.56985151009392,73.000000018974,140.812519108447));
#45130=CARTESIAN_POINT('',(-4.70818579727265,72.500000018974,123.914761837919));
#45131=CARTESIAN_POINT('',(-6.56985151009392,72.500000018974,140.812519108447));
#45132=CARTESIAN_POINT('Origin',(-4.70818579727265,73.000000018974,123.914761837919));
#45133=CARTESIAN_POINT('Origin',(-23.9646016415205,72.500000018974,138.89609852172));
#45134=CARTESIAN_POINT('',(-23.4676087806226,72.500000018974,138.950853395626));
#45135=CARTESIAN_POINT('',(-23.9646016415205,72.500000018974,138.89609852172));
#45136=CARTESIAN_POINT('',(-21.6059430678014,72.500000018974,122.053096125097));
#45137=CARTESIAN_POINT('',(-23.4676087806226,72.500000018974,138.950853395626));
#45138=CARTESIAN_POINT('',(-22.1029359286993,72.500000018974,121.998341251191));
#45139=CARTESIAN_POINT('Origin',(-23.4676087806226,73.000000018974,138.950853395626));
#45140=CARTESIAN_POINT('',(-23.9646016415205,73.000000018974,138.89609852172));
#45141=CARTESIAN_POINT('Origin',(-23.4676087806226,73.000000018974,138.950853395626));
#45142=CARTESIAN_POINT('',(-22.1029359286993,73.000000018974,121.998341251191));
#45143=CARTESIAN_POINT('',(-23.9646016415205,73.000000018974,138.89609852172));
#45144=CARTESIAN_POINT('Origin',(-21.6059430678014,73.000000018974,122.053096125097));
#45145=CARTESIAN_POINT('Origin',(-23.9646016415205,90.500000018974,138.89609852172));
#45146=CARTESIAN_POINT('',(-22.1029359286993,90.000000018974,121.998341251191));
#45147=CARTESIAN_POINT('',(-22.1029359286993,90.500000018974,121.998341251191));
#45148=CARTESIAN_POINT('',(-23.9646016415205,90.000000018974,138.89609852172));
#45149=CARTESIAN_POINT('',(-23.9646016415205,90.500000018974,138.89609852172));
#45150=CARTESIAN_POINT('',(-23.9646016415205,90.000000018974,138.89609852172));
#45151=CARTESIAN_POINT('Origin',(-15.0187301453583,81.500000018974,139.881686252037));
#45152=CARTESIAN_POINT('',(-6.56985151009392,90.500000018974,140.812519108447));
#45153=CARTESIAN_POINT('Origin',(-6.56985151009392,90.000000018974,140.812519108447));
#45154=CARTESIAN_POINT('',(-23.4676087806226,90.500000018974,138.950853395626));
#45155=CARTESIAN_POINT('',(-6.07285864919602,90.500000018974,140.867273982354));
#45156=CARTESIAN_POINT('Origin',(-23.4676087806226,90.000000018974,138.950853395626));
#45157=CARTESIAN_POINT('Origin',(-23.4676087806226,90.000000018974,138.950853395626));
#45158=CARTESIAN_POINT('',(-21.6059430678014,90.500000018974,122.053096125097));
#45159=CARTESIAN_POINT('',(-23.4676087806226,90.500000018974,138.950853395626));
#45160=CARTESIAN_POINT('Origin',(-21.6059430678014,90.000000018974,122.053096125097));
#45161=CARTESIAN_POINT('Origin',(-13.157064432537,81.500000018974,122.983928981508));
#45162=CARTESIAN_POINT('',(-4.70818579727265,90.500000018974,123.914761837919));
#45163=CARTESIAN_POINT('',(-4.21119293637475,90.500000018974,123.969516711825));
#45164=CARTESIAN_POINT('Origin',(-4.70818579727265,90.000000018974,123.914761837919));
#45165=CARTESIAN_POINT('',(-4.9566822277216,87.500000018974,123.887384400965));
#45166=CARTESIAN_POINT('',(-21.3574466373524,87.500000018974,122.080473562051));
#45167=CARTESIAN_POINT('',(-4.9566822277216,87.500000018974,123.887384400965));
#45168=CARTESIAN_POINT('Origin',(-6.07285864919602,90.500000018974,140.867273982354));
#45169=CARTESIAN_POINT('',(-6.56985151009392,90.500000018974,140.812519108447));
#45170=CARTESIAN_POINT('Origin',(-20.8098978982873,87.500000018974,117.110544953072));
#45171=CARTESIAN_POINT('',(-4.40913348865652,87.500000018974,118.917455791986));
#45172=CARTESIAN_POINT('',(-4.40913348865652,87.500000018974,118.917455791986));
#45173=CARTESIAN_POINT('',(-20.8098978982873,87.500000018974,117.110544953072));
#45174=CARTESIAN_POINT('Origin',(-12.6095156934719,81.500000018974,118.014000372529));
#45175=CARTESIAN_POINT('',(-4.40913348865652,87.500000018974,118.917455791986));
#45176=CARTESIAN_POINT('Origin',(-4.40913348865652,87.500000018974,118.917455791986));
#45177=CARTESIAN_POINT('Origin',(-6.56985151009392,90.000000018974,140.812519108447));
#62954=UNCERTAINTY_MEASURE_WITH_UNIT(LENGTH_MEASURE(0.01),#62975,
'DISTANCE_ACCURACY_VALUE',
'Maximum model space distance between geometric entities at asserted c
onnectivities');
#62960=UNCERTAINTY_MEASURE_WITH_UNIT(LENGTH_MEASURE(0.01),#62975,
'DISTANCE_ACCURACY_VALUE',
'Maximum model space distance between geometric entities at asserted c
onnectivities');
#62968=(
GEOMETRIC_REPRESENTATION_CONTEXT(3)
GLOBAL_UNCERTAINTY_ASSIGNED_CONTEXT((#62954))
GLOBAL_UNIT_ASSIGNED_CONTEXT((#62975,#62977,#62978))
REPRESENTATION_CONTEXT('','3D')
);
#62974=(
GEOMETRIC_REPRESENTATION_CONTEXT(3)
GLOBAL_UNCERTAINTY_ASSIGNED_CONTEXT((#62960))
GLOBAL_UNIT_ASSIGNED_CONTEXT((#62975,#62977,#62978))
REPRESENTATION_CONTEXT('','3D')
);
#62975=(
LENGTH_UNIT()
NAMED_UNIT(*)
SI_UNIT(.MILLI.,.METRE.)
);
#62977=(
NAMED_UNIT(*)
PLANE_ANGLE_UNIT()
SI_UNIT($,.RADIAN.)
);
#62978=(
NAMED_UNIT(*)
SI_UNIT($,.STERADIAN.)
SOLID_ANGLE_UNIT()
);
#62986=SHAPE_DEFINITION_REPRESENTATION(#62999,#63027);
#62999=PRODUCT_DEFINITION_SHAPE('',$,#63041);
#63027=SHAPE_REPRESENTATION('',(#16214),#62968);
#63033=PRODUCT_DEFINITION_CONTEXT('part definition',#63074,'design');
#63041=PRODUCT_DEFINITION('MAP Sensor & Vacuum Tube',
'MAP Sensor & Vacuum Tube',#63054,#63033);
#63054=PRODUCT_DEFINITION_FORMATION('',$,#63083);
#63074=APPLICATION_CONTEXT(
'Core Data for Automotive Mechanical Design Process');
#63075=PRODUCT_CONTEXT('part definition',#63074,'mechanical');
#63083=PRODUCT('MAP Sensor & Vacuum Tube','MAP Sensor & Vacuum Tube',$,
(#63075));
#63090=PRESENTATION_STYLE_ASSIGNMENT((#63092));
#63092=SURFACE_STYLE_USAGE(.BOTH.,#63094);
#63094=SURFACE_SIDE_STYLE('',(#63096));
#63096=SURFACE_STYLE_FILL_AREA(#63098);
#63098=FILL_AREA_STYLE('Opaque(202,209,238)',(#63100));
#63100=FILL_AREA_STYLE_COLOUR('Opaque(202,209,238)',#63102);
#63102=COLOUR_RGB('Opaque(202,209,238)', 0.66274510, 0.83137255, 0.94901961);
ENDSEC;
END-ISO-10303-21;
